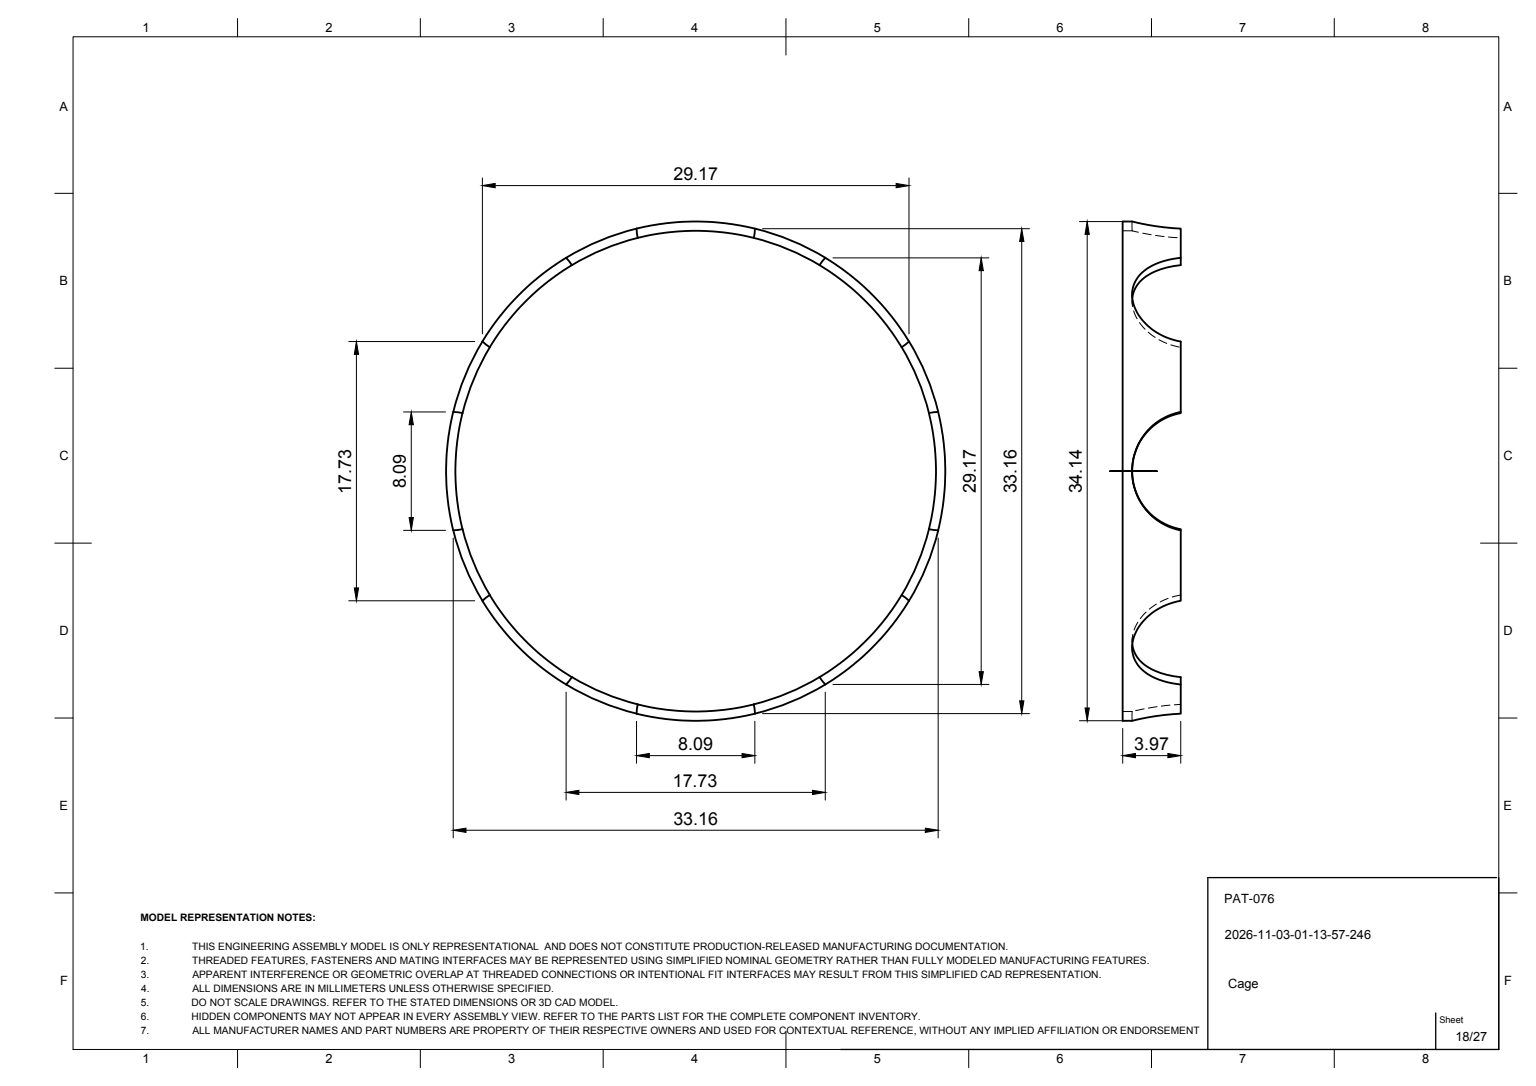
ISO-10303-21;
HEADER;
/* Generated by software containing ST-Developer
 * from STEP Tools, Inc. (www.steptools.com) 
 */

FILE_DESCRIPTION(
/* description */ ('Overhung pulley bearing cartridge'),
/* implementation_level */ '2;1');

FILE_NAME(
/* name */ 'Cage.step',
/* time_stamp */ '2026-10-28T03:22:33-07:00',
/* author */ (''),
/* organization */ (''),
/* preprocessor_version */ 'ST-DEVELOPER v20.2',
/* originating_system */ 'Autodesk Translation Framework v15.17.0.0',
/* authorisation */ '');

FILE_SCHEMA (('AUTOMOTIVE_DESIGN { 1 0 10303 214 3 1 1 }'));
ENDSEC;

DATA;
#10=MECHANICAL_DESIGN_GEOMETRIC_PRESENTATION_REPRESENTATION('',(#301),#10963);
#163=B_SPLINE_CURVE_WITH_KNOTS('',3,(#9085,#9086,#9087,#9088,#9089,#9090,
#9091,#9092,#9093,#9094,#9095,#9096,#9097,#9098,#9099,#9100,#9101,#9102,
#9103,#9104,#9105,#9106),.UNSPECIFIED.,.F.,.F.,(4,2,2,2,2,2,2,2,2,2,4),
(0.0789094028588958,0.210573405340968,0.315860108011452,0.421146810681936,
0.522142632548711,0.623138454415485,0.72413427628226,0.825130098149035,
0.930416800819519,1.03570350349,1.16736750597208),.UNSPECIFIED.);
#164=B_SPLINE_CURVE_WITH_KNOTS('',3,(#9110,#9111,#9112,#9113,#9114,#9115,
#9116,#9117,#9118,#9119,#9120,#9121,#9122,#9123,#9124,#9125,#9126,#9127,
#9128,#9129,#9130,#9131),.UNSPECIFIED.,.F.,.F.,(4,2,2,2,2,2,2,2,2,2,4),
(0.0774793363974613,0.142088896491891,0.284177792983782,0.411119756996526,
0.514392970548519,0.617666184100513,0.720939397652506,0.8242126112045,0.951154575217244,
1.09324347170913,1.15785303180356),.UNSPECIFIED.);
#165=B_SPLINE_CURVE_WITH_KNOTS('',3,(#9137,#9138,#9139,#9140,#9141,#9142,
#9143,#9144,#9145,#9146,#9147,#9148,#9149,#9150,#9151,#9152,#9153,#9154,
#9155,#9156,#9157,#9158),.UNSPECIFIED.,.F.,.F.,(4,2,2,2,2,2,2,2,2,2,4),
(0.0774793363974613,0.142088896491891,0.284177792983782,0.411119756996525,
0.514392970548519,0.617666184100513,0.720939397652506,0.8242126112045,0.951154575217243,
1.09324347170913,1.15785303180356),.UNSPECIFIED.);
#166=B_SPLINE_CURVE_WITH_KNOTS('',3,(#9162,#9163,#9164,#9165,#9166,#9167,
#9168,#9169,#9170,#9171,#9172,#9173,#9174,#9175,#9176,#9177,#9178,#9179,
#9180,#9181,#9182,#9183),.UNSPECIFIED.,.F.,.F.,(4,2,2,2,2,2,2,2,2,2,4),
(0.0774793363974614,0.142088896491891,0.284177792983781,0.411119756996525,
0.514392970548519,0.617666184100512,0.720939397652506,0.824212611204499,
0.951154575217243,1.09324347170913,1.15785303180356),.UNSPECIFIED.);
#167=B_SPLINE_CURVE_WITH_KNOTS('',3,(#9187,#9188,#9189,#9190,#9191,#9192,
#9193,#9194,#9195,#9196,#9197,#9198),.UNSPECIFIED.,.F.,.F.,(4,2,2,2,2,4),
(0.0774793363974613,0.142088896491891,0.284177792983781,0.411119756996525,
0.514392970548519,0.617666184100512),.UNSPECIFIED.);
#168=B_SPLINE_CURVE_WITH_KNOTS('',3,(#9203,#9204,#9205,#9206,#9207,#9208,
#9209,#9210,#9211,#9212,#9213,#9214),.UNSPECIFIED.,.F.,.F.,(4,2,2,2,2,4),
(0.617666184100512,0.720939397652506,0.824212611204499,0.951154575217243,
1.09324347170913,1.15785303180356),.UNSPECIFIED.);
#169=B_SPLINE_CURVE_WITH_KNOTS('',3,(#9218,#9219,#9220,#9221,#9222,#9223,
#9224,#9225,#9226,#9227,#9228,#9229,#9230,#9231,#9232,#9233,#9234,#9235,
#9236,#9237,#9238,#9239),.UNSPECIFIED.,.F.,.F.,(4,2,2,2,2,2,2,2,2,2,4),
(0.0774793363974613,0.142088896491891,0.284177792983782,0.411119756996526,
0.514392970548519,0.617666184100513,0.720939397652507,0.8242126112045,0.951154575217245,
1.09324347170914,1.15785303180356),.UNSPECIFIED.);
#170=B_SPLINE_CURVE_WITH_KNOTS('',3,(#9243,#9244,#9245,#9246,#9247,#9248,
#9249,#9250,#9251,#9252,#9253,#9254,#9255,#9256,#9257,#9258,#9259,#9260,
#9261,#9262,#9263,#9264),.UNSPECIFIED.,.F.,.F.,(4,2,2,2,2,2,2,2,2,2,4),
(0.0774793363974613,0.142088896491891,0.284177792983782,0.411119756996526,
0.514392970548519,0.617666184100513,0.720939397652506,0.824212611204499,
0.951154575217243,1.09324347170913,1.15785303180356),.UNSPECIFIED.);
#171=B_SPLINE_CURVE_WITH_KNOTS('',3,(#9268,#9269,#9270,#9271,#9272,#9273,
#9274,#9275,#9276,#9277,#9278,#9279,#9280,#9281,#9282,#9283,#9284,#9285,
#9286,#9287,#9288,#9289),.UNSPECIFIED.,.F.,.F.,(4,2,2,2,2,2,2,2,2,2,4),
(0.0774793363974613,0.142088896491891,0.284177792983782,0.411119756996526,
0.514392970548519,0.617666184100513,0.720939397652506,0.8242126112045,0.951154575217244,
1.09324347170913,1.15785303180356),.UNSPECIFIED.);
#172=B_SPLINE_CURVE_WITH_KNOTS('',3,(#9293,#9294,#9295,#9296,#9297,#9298,
#9299,#9300,#9301,#9302,#9303,#9304,#9305,#9306,#9307,#9308,#9309,#9310,
#9311,#9312,#9313,#9314),.UNSPECIFIED.,.F.,.F.,(4,2,2,2,2,2,2,2,2,2,4),
(0.0774793363974613,0.142088896491891,0.284177792983782,0.411119756996526,
0.514392970548519,0.617666184100513,0.720939397652506,0.8242126112045,0.951154575217243,
1.09324347170913,1.15785303180356),.UNSPECIFIED.);
#173=B_SPLINE_CURVE_WITH_KNOTS('',3,(#9322,#9323,#9324,#9325,#9326,#9327,
#9328,#9329,#9330,#9331,#9332,#9333,#9334,#9335,#9336,#9337,#9338,#9339,
#9340,#9341,#9342,#9343),.UNSPECIFIED.,.F.,.F.,(4,2,2,2,2,2,2,2,2,2,4),
(0.0789094028588958,0.210573405340968,0.315860108011452,0.421146810681936,
0.522142632548711,0.623138454415485,0.72413427628226,0.825130098149035,
0.930416800819519,1.03570350349,1.16736750597208),.UNSPECIFIED.);
#174=B_SPLINE_CURVE_WITH_KNOTS('',3,(#9351,#9352,#9353,#9354,#9355,#9356,
#9357,#9358,#9359,#9360,#9361,#9362,#9363,#9364,#9365,#9366,#9367,#9368,
#9369,#9370,#9371,#9372),.UNSPECIFIED.,.F.,.F.,(4,2,2,2,2,2,2,2,2,2,4),
(0.0789094028588958,0.210573405340969,0.315860108011453,0.421146810681937,
0.522142632548712,0.623138454415486,0.724134276282261,0.825130098149035,
0.930416800819519,1.03570350349,1.16736750597208),.UNSPECIFIED.);
#175=B_SPLINE_CURVE_WITH_KNOTS('',3,(#9381,#9382,#9383,#9384,#9385,#9386,
#9387,#9388,#9389,#9390,#9391,#9392),.UNSPECIFIED.,.F.,.F.,(4,2,2,2,2,4),
(0.0789094028588958,0.210573405340968,0.315860108011452,0.421146810681937,
0.522142632548711,0.623138454415486),.UNSPECIFIED.);
#176=B_SPLINE_CURVE_WITH_KNOTS('',3,(#9394,#9395,#9396,#9397,#9398,#9399,
#9400,#9401,#9402,#9403,#9404,#9405),.UNSPECIFIED.,.F.,.F.,(4,2,2,2,2,4),
(0.623138454415486,0.72413427628226,0.825130098149035,0.930416800819519,
1.03570350349,1.16736750597208),.UNSPECIFIED.);
#177=B_SPLINE_CURVE_WITH_KNOTS('',3,(#9412,#9413,#9414,#9415,#9416,#9417,
#9418,#9419,#9420,#9421,#9422,#9423,#9424,#9425,#9426,#9427,#9428,#9429,
#9430,#9431,#9432,#9433),.UNSPECIFIED.,.F.,.F.,(4,2,2,2,2,2,2,2,2,2,4),
(0.0789094028588958,0.210573405340968,0.315860108011452,0.421146810681936,
0.522142632548711,0.623138454415486,0.72413427628226,0.825130098149035,
0.930416800819519,1.03570350349,1.16736750597208),.UNSPECIFIED.);
#178=B_SPLINE_CURVE_WITH_KNOTS('',3,(#9441,#9442,#9443,#9444,#9445,#9446,
#9447,#9448,#9449,#9450,#9451,#9452,#9453,#9454,#9455,#9456,#9457,#9458,
#9459,#9460,#9461,#9462),.UNSPECIFIED.,.F.,.F.,(4,2,2,2,2,2,2,2,2,2,4),
(0.0789094028588957,0.210573405340968,0.315860108011452,0.421146810681936,
0.522142632548711,0.623138454415485,0.72413427628226,0.825130098149035,
0.930416800819519,1.03570350349,1.16736750597207),.UNSPECIFIED.);
#179=B_SPLINE_CURVE_WITH_KNOTS('',3,(#9470,#9471,#9472,#9473,#9474,#9475,
#9476,#9477,#9478,#9479,#9480,#9481,#9482,#9483,#9484,#9485,#9486,#9487,
#9488,#9489,#9490,#9491),.UNSPECIFIED.,.F.,.F.,(4,2,2,2,2,2,2,2,2,2,4),
(0.0789094028588958,0.210573405340968,0.315860108011452,0.421146810681936,
0.522142632548711,0.623138454415486,0.72413427628226,0.825130098149035,
0.930416800819519,1.03570350349,1.16736750597208),.UNSPECIFIED.);
#180=B_SPLINE_CURVE_WITH_KNOTS('',3,(#9500,#9501,#9502,#9503,#9504,#9505,
#9506,#9507,#9508,#9509,#9510,#9511,#9512,#9513,#9514,#9515,#9516,#9517,
#9518,#9519,#9520,#9521),.UNSPECIFIED.,.F.,.F.,(4,2,2,2,2,2,2,2,2,2,4),
(0.0789094028588958,0.210573405340968,0.315860108011452,0.421146810681936,
0.522142632548711,0.623138454415485,0.72413427628226,0.825130098149035,
0.930416800819519,1.03570350349,1.16736750597208),.UNSPECIFIED.);
#215=SPHERICAL_SURFACE('',#6170,0.412776);
#216=SPHERICAL_SURFACE('',#6186,0.412776);
#217=SPHERICAL_SURFACE('',#6191,0.412776);
#218=SPHERICAL_SURFACE('',#6196,0.412776);
#219=SPHERICAL_SURFACE('',#6201,0.412776);
#220=SPHERICAL_SURFACE('',#6206,0.412776);
#221=SPHERICAL_SURFACE('',#6211,0.412776);
#222=SPHERICAL_SURFACE('',#6219,0.412776);
#250=SHAPE_REPRESENTATION_RELATIONSHIP('SRR','None',#11071,#272);
#272=ADVANCED_BREP_SHAPE_REPRESENTATION('',(#331),#10951);
#301=STYLED_ITEM('',(#11253),#331);
#331=MANIFOLD_SOLID_BREP('Continuous crown cage',#5668);
#400=FACE_BOUND('',#1101,.T.);
#495=PLANE('',#6183);
#496=PLANE('',#6188);
#497=PLANE('',#6193);
#498=PLANE('',#6198);
#499=PLANE('',#6203);
#500=PLANE('',#6208);
#501=PLANE('',#6217);
#502=PLANE('',#6221);
#503=PLANE('',#6222);
#695=FACE_OUTER_BOUND('',#1083,.T.);
#696=FACE_OUTER_BOUND('',#1084,.T.);
#697=FACE_OUTER_BOUND('',#1085,.T.);
#698=FACE_OUTER_BOUND('',#1086,.T.);
#699=FACE_OUTER_BOUND('',#1087,.T.);
#700=FACE_OUTER_BOUND('',#1088,.T.);
#701=FACE_OUTER_BOUND('',#1089,.T.);
#702=FACE_OUTER_BOUND('',#1090,.T.);
#703=FACE_OUTER_BOUND('',#1091,.T.);
#704=FACE_OUTER_BOUND('',#1092,.T.);
#705=FACE_OUTER_BOUND('',#1093,.T.);
#706=FACE_OUTER_BOUND('',#1094,.T.);
#707=FACE_OUTER_BOUND('',#1095,.T.);
#708=FACE_OUTER_BOUND('',#1096,.T.);
#709=FACE_OUTER_BOUND('',#1097,.T.);
#710=FACE_OUTER_BOUND('',#1098,.T.);
#711=FACE_OUTER_BOUND('',#1099,.T.);
#712=FACE_OUTER_BOUND('',#1100,.T.);
#713=FACE_OUTER_BOUND('',#1102,.T.);
#1083=EDGE_LOOP('',(#4115,#4116,#4117,#4118));
#1084=EDGE_LOOP('',(#4119,#4120,#4121,#4122,#4123,#4124,#4125,#4126,#4127,
#4128,#4129,#4130,#4131,#4132,#4133,#4134,#4135,#4136,#4137,#4138));
#1085=EDGE_LOOP('',(#4139,#4140,#4141,#4142));
#1086=EDGE_LOOP('',(#4143,#4144,#4145,#4146));
#1087=EDGE_LOOP('',(#4147,#4148,#4149,#4150));
#1088=EDGE_LOOP('',(#4151,#4152,#4153,#4154));
#1089=EDGE_LOOP('',(#4155,#4156,#4157,#4158));
#1090=EDGE_LOOP('',(#4159,#4160,#4161,#4162,#4163,#4164));
#1091=EDGE_LOOP('',(#4165,#4166,#4167,#4168));
#1092=EDGE_LOOP('',(#4169,#4170,#4171,#4172));
#1093=EDGE_LOOP('',(#4173,#4174,#4175,#4176));
#1094=EDGE_LOOP('',(#4177,#4178,#4179,#4180));
#1095=EDGE_LOOP('',(#4181,#4182,#4183,#4184));
#1096=EDGE_LOOP('',(#4185,#4186,#4187,#4188));
#1097=EDGE_LOOP('',(#4189,#4190,#4191,#4192,#4193,#4194,#4195,#4196,#4197,
#4198,#4199,#4200,#4201,#4202,#4203,#4204,#4205,#4206,#4207,#4208));
#1098=EDGE_LOOP('',(#4209,#4210,#4211,#4212));
#1099=EDGE_LOOP('',(#4213,#4214,#4215,#4216));
#1100=EDGE_LOOP('',(#4217));
#1101=EDGE_LOOP('',(#4218));
#1102=EDGE_LOOP('',(#4219,#4220,#4221,#4222));
#1447=LINE('',#9200,#1789);
#1448=LINE('',#9496,#1790);
#1789=VECTOR('',#7311,1.706752);
#1790=VECTOR('',#7388,1.643248);
#2124=CIRCLE('',#6171,0.405071403305639);
#2125=CIRCLE('',#6172,0.405071403305639);
#2126=CIRCLE('',#6174,1.706752);
#2127=CIRCLE('',#6175,1.706752);
#2128=CIRCLE('',#6176,1.706752);
#2129=CIRCLE('',#6177,1.706752);
#2130=CIRCLE('',#6178,1.706752);
#2131=CIRCLE('',#6179,1.706752);
#2132=CIRCLE('',#6180,1.706752);
#2133=CIRCLE('',#6181,1.706752);
#2134=CIRCLE('',#6182,1.706752);
#2135=CIRCLE('',#6184,1.643248);
#2136=CIRCLE('',#6185,0.405071403305639);
#2137=CIRCLE('',#6187,0.405071403305639);
#2138=CIRCLE('',#6189,1.643248);
#2139=CIRCLE('',#6190,0.405071403305639);
#2140=CIRCLE('',#6192,0.405071403305639);
#2141=CIRCLE('',#6194,1.643248);
#2142=CIRCLE('',#6195,0.405071403305639);
#2143=CIRCLE('',#6197,0.405071403305639);
#2144=CIRCLE('',#6199,1.643248);
#2145=CIRCLE('',#6200,0.405071403305639);
#2146=CIRCLE('',#6202,0.405071403305639);
#2147=CIRCLE('',#6204,1.643248);
#2148=CIRCLE('',#6205,0.405071403305639);
#2149=CIRCLE('',#6207,0.405071403305639);
#2150=CIRCLE('',#6209,1.643248);
#2151=CIRCLE('',#6210,0.405071403305639);
#2152=CIRCLE('',#6212,0.405071403305639);
#2153=CIRCLE('',#6214,1.643248);
#2154=CIRCLE('',#6215,1.643248);
#2155=CIRCLE('',#6216,1.643248);
#2156=CIRCLE('',#6218,0.405071403305639);
#2157=CIRCLE('',#6220,0.405071403305639);
#2545=VERTEX_POINT('',#9083);
#2546=VERTEX_POINT('',#9084);
#2547=VERTEX_POINT('',#9107);
#2548=VERTEX_POINT('',#9109);
#2549=VERTEX_POINT('',#9134);
#2550=VERTEX_POINT('',#9136);
#2551=VERTEX_POINT('',#9159);
#2552=VERTEX_POINT('',#9161);
#2553=VERTEX_POINT('',#9184);
#2554=VERTEX_POINT('',#9186);
#2555=VERTEX_POINT('',#9199);
#2556=VERTEX_POINT('',#9202);
#2557=VERTEX_POINT('',#9215);
#2558=VERTEX_POINT('',#9217);
#2559=VERTEX_POINT('',#9240);
#2560=VERTEX_POINT('',#9242);
#2561=VERTEX_POINT('',#9265);
#2562=VERTEX_POINT('',#9267);
#2563=VERTEX_POINT('',#9290);
#2564=VERTEX_POINT('',#9292);
#2565=VERTEX_POINT('',#9317);
#2566=VERTEX_POINT('',#9321);
#2567=VERTEX_POINT('',#9346);
#2568=VERTEX_POINT('',#9350);
#2569=VERTEX_POINT('',#9375);
#2570=VERTEX_POINT('',#9379);
#2571=VERTEX_POINT('',#9380);
#2572=VERTEX_POINT('',#9407);
#2573=VERTEX_POINT('',#9411);
#2574=VERTEX_POINT('',#9436);
#2575=VERTEX_POINT('',#9440);
#2576=VERTEX_POINT('',#9465);
#2577=VERTEX_POINT('',#9469);
#2578=VERTEX_POINT('',#9494);
#2579=VERTEX_POINT('',#9497);
#2580=VERTEX_POINT('',#9499);
#3127=EDGE_CURVE('',#2545,#2546,#163,.T.);
#3128=EDGE_CURVE('',#2547,#2545,#2124,.T.);
#3129=EDGE_CURVE('',#2548,#2547,#164,.T.);
#3130=EDGE_CURVE('',#2546,#2548,#2125,.T.);
#3131=EDGE_CURVE('',#2549,#2547,#2126,.T.);
#3132=EDGE_CURVE('',#2549,#2550,#165,.T.);
#3133=EDGE_CURVE('',#2551,#2550,#2127,.T.);
#3134=EDGE_CURVE('',#2551,#2552,#166,.T.);
#3135=EDGE_CURVE('',#2553,#2552,#2128,.T.);
#3136=EDGE_CURVE('',#2553,#2554,#167,.T.);
#3137=EDGE_CURVE('',#2554,#2555,#1447,.T.);
#3138=EDGE_CURVE('',#2555,#2555,#2129,.T.);
#3139=EDGE_CURVE('',#2554,#2556,#168,.T.);
#3140=EDGE_CURVE('',#2557,#2556,#2130,.T.);
#3141=EDGE_CURVE('',#2557,#2558,#169,.T.);
#3142=EDGE_CURVE('',#2559,#2558,#2131,.T.);
#3143=EDGE_CURVE('',#2559,#2560,#170,.T.);
#3144=EDGE_CURVE('',#2561,#2560,#2132,.T.);
#3145=EDGE_CURVE('',#2561,#2562,#171,.T.);
#3146=EDGE_CURVE('',#2563,#2562,#2133,.T.);
#3147=EDGE_CURVE('',#2563,#2564,#172,.T.);
#3148=EDGE_CURVE('',#2548,#2564,#2134,.T.);
#3149=EDGE_CURVE('',#2545,#2565,#2135,.T.);
#3150=EDGE_CURVE('',#2565,#2549,#2136,.T.);
#3151=EDGE_CURVE('',#2566,#2565,#173,.T.);
#3152=EDGE_CURVE('',#2550,#2566,#2137,.T.);
#3153=EDGE_CURVE('',#2566,#2567,#2138,.T.);
#3154=EDGE_CURVE('',#2567,#2551,#2139,.T.);
#3155=EDGE_CURVE('',#2568,#2567,#174,.T.);
#3156=EDGE_CURVE('',#2552,#2568,#2140,.T.);
#3157=EDGE_CURVE('',#2568,#2569,#2141,.T.);
#3158=EDGE_CURVE('',#2569,#2553,#2142,.T.);
#3159=EDGE_CURVE('',#2570,#2571,#175,.T.);
#3160=EDGE_CURVE('',#2556,#2570,#2143,.T.);
#3161=EDGE_CURVE('',#2571,#2569,#176,.T.);
#3162=EDGE_CURVE('',#2570,#2572,#2144,.T.);
#3163=EDGE_CURVE('',#2572,#2557,#2145,.T.);
#3164=EDGE_CURVE('',#2573,#2572,#177,.T.);
#3165=EDGE_CURVE('',#2558,#2573,#2146,.T.);
#3166=EDGE_CURVE('',#2573,#2574,#2147,.T.);
#3167=EDGE_CURVE('',#2574,#2559,#2148,.T.);
#3168=EDGE_CURVE('',#2575,#2574,#178,.T.);
#3169=EDGE_CURVE('',#2560,#2575,#2149,.T.);
#3170=EDGE_CURVE('',#2575,#2576,#2150,.T.);
#3171=EDGE_CURVE('',#2576,#2561,#2151,.T.);
#3172=EDGE_CURVE('',#2577,#2576,#179,.T.);
#3173=EDGE_CURVE('',#2562,#2577,#2152,.T.);
#3174=EDGE_CURVE('',#2578,#2578,#2153,.T.);
#3175=EDGE_CURVE('',#2578,#2571,#1448,.T.);
#3176=EDGE_CURVE('',#2579,#2546,#2154,.T.);
#3177=EDGE_CURVE('',#2579,#2580,#180,.T.);
#3178=EDGE_CURVE('',#2577,#2580,#2155,.T.);
#3179=EDGE_CURVE('',#2564,#2579,#2156,.T.);
#3180=EDGE_CURVE('',#2580,#2563,#2157,.T.);
#4115=ORIENTED_EDGE('',*,*,#3127,.F.);
#4116=ORIENTED_EDGE('',*,*,#3128,.F.);
#4117=ORIENTED_EDGE('',*,*,#3129,.F.);
#4118=ORIENTED_EDGE('',*,*,#3130,.F.);
#4119=ORIENTED_EDGE('',*,*,#3129,.T.);
#4120=ORIENTED_EDGE('',*,*,#3131,.F.);
#4121=ORIENTED_EDGE('',*,*,#3132,.T.);
#4122=ORIENTED_EDGE('',*,*,#3133,.F.);
#4123=ORIENTED_EDGE('',*,*,#3134,.T.);
#4124=ORIENTED_EDGE('',*,*,#3135,.F.);
#4125=ORIENTED_EDGE('',*,*,#3136,.T.);
#4126=ORIENTED_EDGE('',*,*,#3137,.T.);
#4127=ORIENTED_EDGE('',*,*,#3138,.F.);
#4128=ORIENTED_EDGE('',*,*,#3137,.F.);
#4129=ORIENTED_EDGE('',*,*,#3139,.T.);
#4130=ORIENTED_EDGE('',*,*,#3140,.F.);
#4131=ORIENTED_EDGE('',*,*,#3141,.T.);
#4132=ORIENTED_EDGE('',*,*,#3142,.F.);
#4133=ORIENTED_EDGE('',*,*,#3143,.T.);
#4134=ORIENTED_EDGE('',*,*,#3144,.F.);
#4135=ORIENTED_EDGE('',*,*,#3145,.T.);
#4136=ORIENTED_EDGE('',*,*,#3146,.F.);
#4137=ORIENTED_EDGE('',*,*,#3147,.T.);
#4138=ORIENTED_EDGE('',*,*,#3148,.F.);
#4139=ORIENTED_EDGE('',*,*,#3128,.T.);
#4140=ORIENTED_EDGE('',*,*,#3149,.T.);
#4141=ORIENTED_EDGE('',*,*,#3150,.T.);
#4142=ORIENTED_EDGE('',*,*,#3131,.T.);
#4143=ORIENTED_EDGE('',*,*,#3151,.F.);
#4144=ORIENTED_EDGE('',*,*,#3152,.F.);
#4145=ORIENTED_EDGE('',*,*,#3132,.F.);
#4146=ORIENTED_EDGE('',*,*,#3150,.F.);
#4147=ORIENTED_EDGE('',*,*,#3152,.T.);
#4148=ORIENTED_EDGE('',*,*,#3153,.T.);
#4149=ORIENTED_EDGE('',*,*,#3154,.T.);
#4150=ORIENTED_EDGE('',*,*,#3133,.T.);
#4151=ORIENTED_EDGE('',*,*,#3155,.F.);
#4152=ORIENTED_EDGE('',*,*,#3156,.F.);
#4153=ORIENTED_EDGE('',*,*,#3134,.F.);
#4154=ORIENTED_EDGE('',*,*,#3154,.F.);
#4155=ORIENTED_EDGE('',*,*,#3156,.T.);
#4156=ORIENTED_EDGE('',*,*,#3157,.T.);
#4157=ORIENTED_EDGE('',*,*,#3158,.T.);
#4158=ORIENTED_EDGE('',*,*,#3135,.T.);
#4159=ORIENTED_EDGE('',*,*,#3159,.F.);
#4160=ORIENTED_EDGE('',*,*,#3160,.F.);
#4161=ORIENTED_EDGE('',*,*,#3139,.F.);
#4162=ORIENTED_EDGE('',*,*,#3136,.F.);
#4163=ORIENTED_EDGE('',*,*,#3158,.F.);
#4164=ORIENTED_EDGE('',*,*,#3161,.F.);
#4165=ORIENTED_EDGE('',*,*,#3160,.T.);
#4166=ORIENTED_EDGE('',*,*,#3162,.T.);
#4167=ORIENTED_EDGE('',*,*,#3163,.T.);
#4168=ORIENTED_EDGE('',*,*,#3140,.T.);
#4169=ORIENTED_EDGE('',*,*,#3164,.F.);
#4170=ORIENTED_EDGE('',*,*,#3165,.F.);
#4171=ORIENTED_EDGE('',*,*,#3141,.F.);
#4172=ORIENTED_EDGE('',*,*,#3163,.F.);
#4173=ORIENTED_EDGE('',*,*,#3165,.T.);
#4174=ORIENTED_EDGE('',*,*,#3166,.T.);
#4175=ORIENTED_EDGE('',*,*,#3167,.T.);
#4176=ORIENTED_EDGE('',*,*,#3142,.T.);
#4177=ORIENTED_EDGE('',*,*,#3168,.F.);
#4178=ORIENTED_EDGE('',*,*,#3169,.F.);
#4179=ORIENTED_EDGE('',*,*,#3143,.F.);
#4180=ORIENTED_EDGE('',*,*,#3167,.F.);
#4181=ORIENTED_EDGE('',*,*,#3169,.T.);
#4182=ORIENTED_EDGE('',*,*,#3170,.T.);
#4183=ORIENTED_EDGE('',*,*,#3171,.T.);
#4184=ORIENTED_EDGE('',*,*,#3144,.T.);
#4185=ORIENTED_EDGE('',*,*,#3145,.F.);
#4186=ORIENTED_EDGE('',*,*,#3171,.F.);
#4187=ORIENTED_EDGE('',*,*,#3172,.F.);
#4188=ORIENTED_EDGE('',*,*,#3173,.F.);
#4189=ORIENTED_EDGE('',*,*,#3174,.F.);
#4190=ORIENTED_EDGE('',*,*,#3175,.T.);
#4191=ORIENTED_EDGE('',*,*,#3161,.T.);
#4192=ORIENTED_EDGE('',*,*,#3157,.F.);
#4193=ORIENTED_EDGE('',*,*,#3155,.T.);
#4194=ORIENTED_EDGE('',*,*,#3153,.F.);
#4195=ORIENTED_EDGE('',*,*,#3151,.T.);
#4196=ORIENTED_EDGE('',*,*,#3149,.F.);
#4197=ORIENTED_EDGE('',*,*,#3127,.T.);
#4198=ORIENTED_EDGE('',*,*,#3176,.F.);
#4199=ORIENTED_EDGE('',*,*,#3177,.T.);
#4200=ORIENTED_EDGE('',*,*,#3178,.F.);
#4201=ORIENTED_EDGE('',*,*,#3172,.T.);
#4202=ORIENTED_EDGE('',*,*,#3170,.F.);
#4203=ORIENTED_EDGE('',*,*,#3168,.T.);
#4204=ORIENTED_EDGE('',*,*,#3166,.F.);
#4205=ORIENTED_EDGE('',*,*,#3164,.T.);
#4206=ORIENTED_EDGE('',*,*,#3162,.F.);
#4207=ORIENTED_EDGE('',*,*,#3159,.T.);
#4208=ORIENTED_EDGE('',*,*,#3175,.F.);
#4209=ORIENTED_EDGE('',*,*,#3130,.T.);
#4210=ORIENTED_EDGE('',*,*,#3148,.T.);
#4211=ORIENTED_EDGE('',*,*,#3179,.T.);
#4212=ORIENTED_EDGE('',*,*,#3176,.T.);
#4213=ORIENTED_EDGE('',*,*,#3147,.F.);
#4214=ORIENTED_EDGE('',*,*,#3180,.F.);
#4215=ORIENTED_EDGE('',*,*,#3177,.F.);
#4216=ORIENTED_EDGE('',*,*,#3179,.F.);
#4217=ORIENTED_EDGE('',*,*,#3138,.T.);
#4218=ORIENTED_EDGE('',*,*,#3174,.T.);
#4219=ORIENTED_EDGE('',*,*,#3173,.T.);
#4220=ORIENTED_EDGE('',*,*,#3178,.T.);
#4221=ORIENTED_EDGE('',*,*,#3180,.T.);
#4222=ORIENTED_EDGE('',*,*,#3146,.T.);
#5210=CYLINDRICAL_SURFACE('',#6173,1.706752);
#5211=CYLINDRICAL_SURFACE('',#6213,1.643248);
#5439=ADVANCED_FACE('',(#695),#215,.F.);
#5440=ADVANCED_FACE('',(#696),#5210,.T.);
#5441=ADVANCED_FACE('',(#697),#495,.T.);
#5442=ADVANCED_FACE('',(#698),#216,.F.);
#5443=ADVANCED_FACE('',(#699),#496,.T.);
#5444=ADVANCED_FACE('',(#700),#217,.F.);
#5445=ADVANCED_FACE('',(#701),#497,.T.);
#5446=ADVANCED_FACE('',(#702),#218,.F.);
#5447=ADVANCED_FACE('',(#703),#498,.T.);
#5448=ADVANCED_FACE('',(#704),#219,.F.);
#5449=ADVANCED_FACE('',(#705),#499,.T.);
#5450=ADVANCED_FACE('',(#706),#220,.F.);
#5451=ADVANCED_FACE('',(#707),#500,.T.);
#5452=ADVANCED_FACE('',(#708),#221,.F.);
#5453=ADVANCED_FACE('',(#709),#5211,.F.);
#5454=ADVANCED_FACE('',(#710),#501,.T.);
#5455=ADVANCED_FACE('',(#711),#222,.F.);
#5456=ADVANCED_FACE('',(#712,#400),#502,.T.);
#5457=ADVANCED_FACE('',(#713),#503,.T.);
#5668=CLOSED_SHELL('',(#5439,#5440,#5441,#5442,#5443,#5444,#5445,#5446,
#5447,#5448,#5449,#5450,#5451,#5452,#5453,#5454,#5455,#5456,#5457));
#6169=AXIS2_PLACEMENT_3D('',#9081,#7295,#7296);
#6170=AXIS2_PLACEMENT_3D('',#9082,#7297,#7298);
#6171=AXIS2_PLACEMENT_3D('',#9108,#7299,#7300);
#6172=AXIS2_PLACEMENT_3D('',#9132,#7301,#7302);
#6173=AXIS2_PLACEMENT_3D('',#9133,#7303,#7304);
#6174=AXIS2_PLACEMENT_3D('',#9135,#7305,#7306);
#6175=AXIS2_PLACEMENT_3D('',#9160,#7307,#7308);
#6176=AXIS2_PLACEMENT_3D('',#9185,#7309,#7310);
#6177=AXIS2_PLACEMENT_3D('',#9201,#7312,#7313);
#6178=AXIS2_PLACEMENT_3D('',#9216,#7314,#7315);
#6179=AXIS2_PLACEMENT_3D('',#9241,#7316,#7317);
#6180=AXIS2_PLACEMENT_3D('',#9266,#7318,#7319);
#6181=AXIS2_PLACEMENT_3D('',#9291,#7320,#7321);
#6182=AXIS2_PLACEMENT_3D('',#9315,#7322,#7323);
#6183=AXIS2_PLACEMENT_3D('',#9316,#7324,#7325);
#6184=AXIS2_PLACEMENT_3D('',#9318,#7326,#7327);
#6185=AXIS2_PLACEMENT_3D('',#9319,#7328,#7329);
#6186=AXIS2_PLACEMENT_3D('',#9320,#7330,#7331);
#6187=AXIS2_PLACEMENT_3D('',#9344,#7332,#7333);
#6188=AXIS2_PLACEMENT_3D('',#9345,#7334,#7335);
#6189=AXIS2_PLACEMENT_3D('',#9347,#7336,#7337);
#6190=AXIS2_PLACEMENT_3D('',#9348,#7338,#7339);
#6191=AXIS2_PLACEMENT_3D('',#9349,#7340,#7341);
#6192=AXIS2_PLACEMENT_3D('',#9373,#7342,#7343);
#6193=AXIS2_PLACEMENT_3D('',#9374,#7344,#7345);
#6194=AXIS2_PLACEMENT_3D('',#9376,#7346,#7347);
#6195=AXIS2_PLACEMENT_3D('',#9377,#7348,#7349);
#6196=AXIS2_PLACEMENT_3D('',#9378,#7350,#7351);
#6197=AXIS2_PLACEMENT_3D('',#9393,#7352,#7353);
#6198=AXIS2_PLACEMENT_3D('',#9406,#7354,#7355);
#6199=AXIS2_PLACEMENT_3D('',#9408,#7356,#7357);
#6200=AXIS2_PLACEMENT_3D('',#9409,#7358,#7359);
#6201=AXIS2_PLACEMENT_3D('',#9410,#7360,#7361);
#6202=AXIS2_PLACEMENT_3D('',#9434,#7362,#7363);
#6203=AXIS2_PLACEMENT_3D('',#9435,#7364,#7365);
#6204=AXIS2_PLACEMENT_3D('',#9437,#7366,#7367);
#6205=AXIS2_PLACEMENT_3D('',#9438,#7368,#7369);
#6206=AXIS2_PLACEMENT_3D('',#9439,#7370,#7371);
#6207=AXIS2_PLACEMENT_3D('',#9463,#7372,#7373);
#6208=AXIS2_PLACEMENT_3D('',#9464,#7374,#7375);
#6209=AXIS2_PLACEMENT_3D('',#9466,#7376,#7377);
#6210=AXIS2_PLACEMENT_3D('',#9467,#7378,#7379);
#6211=AXIS2_PLACEMENT_3D('',#9468,#7380,#7381);
#6212=AXIS2_PLACEMENT_3D('',#9492,#7382,#7383);
#6213=AXIS2_PLACEMENT_3D('',#9493,#7384,#7385);
#6214=AXIS2_PLACEMENT_3D('',#9495,#7386,#7387);
#6215=AXIS2_PLACEMENT_3D('',#9498,#7389,#7390);
#6216=AXIS2_PLACEMENT_3D('',#9522,#7391,#7392);
#6217=AXIS2_PLACEMENT_3D('',#9523,#7393,#7394);
#6218=AXIS2_PLACEMENT_3D('',#9524,#7395,#7396);
#6219=AXIS2_PLACEMENT_3D('',#9525,#7397,#7398);
#6220=AXIS2_PLACEMENT_3D('',#9526,#7399,#7400);
#6221=AXIS2_PLACEMENT_3D('',#9527,#7401,#7402);
#6222=AXIS2_PLACEMENT_3D('',#9528,#7403,#7404);
#7295=DIRECTION('axis',(0.,0.,1.));
#7296=DIRECTION('refdir',(1.,0.,0.));
#7297=DIRECTION('center_axis',(0.,0.,1.));
#7298=DIRECTION('ref_axis',(1.,0.,0.));
#7299=DIRECTION('center_axis',(0.,-1.,0.));
#7300=DIRECTION('ref_axis',(0.,0.,-1.));
#7301=DIRECTION('center_axis',(0.,-1.,0.));
#7302=DIRECTION('ref_axis',(0.,0.,-1.));
#7303=DIRECTION('center_axis',(0.,1.,0.));
#7304=DIRECTION('ref_axis',(1.,0.,0.));
#7305=DIRECTION('center_axis',(0.,1.,0.));
#7306=DIRECTION('ref_axis',(1.,0.,0.));
#7307=DIRECTION('center_axis',(0.,1.,0.));
#7308=DIRECTION('ref_axis',(1.,0.,0.));
#7309=DIRECTION('center_axis',(0.,1.,0.));
#7310=DIRECTION('ref_axis',(1.,0.,0.));
#7311=DIRECTION('',(0.,-1.,0.));
#7312=DIRECTION('center_axis',(0.,-1.,0.));
#7313=DIRECTION('ref_axis',(1.,0.,0.));
#7314=DIRECTION('center_axis',(0.,1.,0.));
#7315=DIRECTION('ref_axis',(1.,0.,0.));
#7316=DIRECTION('center_axis',(0.,1.,0.));
#7317=DIRECTION('ref_axis',(1.,0.,0.));
#7318=DIRECTION('center_axis',(0.,1.,0.));
#7319=DIRECTION('ref_axis',(1.,0.,0.));
#7320=DIRECTION('center_axis',(0.,1.,0.));
#7321=DIRECTION('ref_axis',(1.,0.,0.));
#7322=DIRECTION('center_axis',(0.,1.,0.));
#7323=DIRECTION('ref_axis',(1.,0.,0.));
#7324=DIRECTION('center_axis',(0.,1.,0.));
#7325=DIRECTION('ref_axis',(1.,0.,0.));
#7326=DIRECTION('center_axis',(0.,-1.,0.));
#7327=DIRECTION('ref_axis',(1.,0.,0.));
#7328=DIRECTION('center_axis',(0.,-1.,0.));
#7329=DIRECTION('ref_axis',(0.,0.,-1.));
#7330=DIRECTION('center_axis',(6.12323399573677E-17,0.,1.));
#7331=DIRECTION('ref_axis',(1.,0.,0.));
#7332=DIRECTION('center_axis',(0.,-1.,0.));
#7333=DIRECTION('ref_axis',(0.,0.,-1.));
#7334=DIRECTION('center_axis',(0.,1.,0.));
#7335=DIRECTION('ref_axis',(1.,0.,0.));
#7336=DIRECTION('center_axis',(0.,-1.,0.));
#7337=DIRECTION('ref_axis',(1.,0.,0.));
#7338=DIRECTION('center_axis',(0.,-1.,0.));
#7339=DIRECTION('ref_axis',(0.,0.,-1.));
#7340=DIRECTION('center_axis',(0.,0.,1.));
#7341=DIRECTION('ref_axis',(1.,0.,0.));
#7342=DIRECTION('center_axis',(0.,-1.,0.));
#7343=DIRECTION('ref_axis',(0.,0.,-1.));
#7344=DIRECTION('center_axis',(0.,1.,0.));
#7345=DIRECTION('ref_axis',(1.,0.,0.));
#7346=DIRECTION('center_axis',(0.,-1.,0.));
#7347=DIRECTION('ref_axis',(1.,0.,0.));
#7348=DIRECTION('center_axis',(0.,-1.,0.));
#7349=DIRECTION('ref_axis',(0.,0.,-1.));
#7350=DIRECTION('center_axis',(0.,0.,1.));
#7351=DIRECTION('ref_axis',(1.,0.,0.));
#7352=DIRECTION('center_axis',(0.,-1.,0.));
#7353=DIRECTION('ref_axis',(0.,0.,-1.));
#7354=DIRECTION('center_axis',(0.,1.,0.));
#7355=DIRECTION('ref_axis',(1.,0.,0.));
#7356=DIRECTION('center_axis',(0.,-1.,0.));
#7357=DIRECTION('ref_axis',(1.,0.,0.));
#7358=DIRECTION('center_axis',(0.,-1.,0.));
#7359=DIRECTION('ref_axis',(0.,0.,-1.));
#7360=DIRECTION('center_axis',(0.,0.,1.));
#7361=DIRECTION('ref_axis',(1.,0.,0.));
#7362=DIRECTION('center_axis',(0.,-1.,0.));
#7363=DIRECTION('ref_axis',(0.,0.,-1.));
#7364=DIRECTION('center_axis',(0.,1.,0.));
#7365=DIRECTION('ref_axis',(1.,0.,0.));
#7366=DIRECTION('center_axis',(0.,-1.,0.));
#7367=DIRECTION('ref_axis',(1.,0.,0.));
#7368=DIRECTION('center_axis',(0.,-1.,0.));
#7369=DIRECTION('ref_axis',(0.,0.,-1.));
#7370=DIRECTION('center_axis',(6.12323399573676E-17,0.,1.));
#7371=DIRECTION('ref_axis',(1.,0.,0.));
#7372=DIRECTION('center_axis',(0.,-1.,0.));
#7373=DIRECTION('ref_axis',(0.,0.,-1.));
#7374=DIRECTION('center_axis',(0.,1.,0.));
#7375=DIRECTION('ref_axis',(1.,0.,0.));
#7376=DIRECTION('center_axis',(0.,-1.,0.));
#7377=DIRECTION('ref_axis',(1.,0.,0.));
#7378=DIRECTION('center_axis',(0.,-1.,0.));
#7379=DIRECTION('ref_axis',(0.,0.,-1.));
#7380=DIRECTION('center_axis',(0.,0.,1.));
#7381=DIRECTION('ref_axis',(1.,0.,0.));
#7382=DIRECTION('center_axis',(0.,-1.,0.));
#7383=DIRECTION('ref_axis',(0.,0.,-1.));
#7384=DIRECTION('center_axis',(0.,1.,0.));
#7385=DIRECTION('ref_axis',(1.,0.,0.));
#7386=DIRECTION('center_axis',(0.,1.,0.));
#7387=DIRECTION('ref_axis',(1.,0.,0.));
#7388=DIRECTION('',(0.,1.,0.));
#7389=DIRECTION('center_axis',(0.,-1.,0.));
#7390=DIRECTION('ref_axis',(1.,0.,0.));
#7391=DIRECTION('center_axis',(0.,-1.,0.));
#7392=DIRECTION('ref_axis',(1.,0.,0.));
#7393=DIRECTION('center_axis',(0.,1.,0.));
#7394=DIRECTION('ref_axis',(1.,0.,0.));
#7395=DIRECTION('center_axis',(0.,-1.,0.));
#7396=DIRECTION('ref_axis',(0.,0.,-1.));
#7397=DIRECTION('center_axis',(0.,0.,1.));
#7398=DIRECTION('ref_axis',(1.,0.,0.));
#7399=DIRECTION('center_axis',(0.,-1.,0.));
#7400=DIRECTION('ref_axis',(0.,0.,-1.));
#7401=DIRECTION('center_axis',(0.,-1.,0.));
#7402=DIRECTION('ref_axis',(-1.,0.,0.));
#7403=DIRECTION('center_axis',(0.,1.,0.));
#7404=DIRECTION('ref_axis',(1.,0.,0.));
#9081=CARTESIAN_POINT('',(0.,0.,0.));
#9082=CARTESIAN_POINT('Origin',(1.18440385848747,0.,1.18440385848747));
#9083=CARTESIAN_POINT('',(0.846804978391753,-0.07938,1.40825612658882));
#9084=CARTESIAN_POINT('',(1.40825612658882,-0.07938,0.846804978391754));
#9085=CARTESIAN_POINT('Ctrl Pts',(0.846804978391752,-0.0793800000000001,
1.40825612658882));
#9086=CARTESIAN_POINT('Ctrl Pts',(0.854205272175554,-0.123401821157026,
1.40380622184538));
#9087=CARTESIAN_POINT('Ctrl Pts',(0.867957148219441,-0.166543350814306,
1.39550172959303));
#9088=CARTESIAN_POINT('Ctrl Pts',(0.902193646979982,-0.237231147975234,
1.3735491215176));
#9089=CARTESIAN_POINT('Ctrl Pts',(0.920778333482564,-0.266264900654909,
1.36127834356734));
#9090=CARTESIAN_POINT('Ctrl Pts',(0.962485392528369,-0.317195968905306,
1.33211611256184));
#9091=CARTESIAN_POINT('Ctrl Pts',(0.985600426557816,-0.33909093068465,1.31521005565926));
#9092=CARTESIAN_POINT('Ctrl Pts',(1.03253285680459,-0.373586846396559,1.27866649102984));
#9093=CARTESIAN_POINT('Ctrl Pts',(1.05871835910697,-0.388086240756494,1.25722555095714));
#9094=CARTESIAN_POINT('Ctrl Pts',(1.11153475808518,-0.407068917407805,1.2107812086231));
#9095=CARTESIAN_POINT('Ctrl Pts',(1.13814686046673,-0.411552957311693,1.18575674747573));
#9096=CARTESIAN_POINT('Ctrl Pts',(1.18575674747573,-0.411552957311693,1.13814686046673));
#9097=CARTESIAN_POINT('Ctrl Pts',(1.2107812086231,-0.407068917407805,1.11153475808518));
#9098=CARTESIAN_POINT('Ctrl Pts',(1.25722555095713,-0.388086240756494,1.05871835910697));
#9099=CARTESIAN_POINT('Ctrl Pts',(1.27866649102984,-0.373586846396559,1.03253285680459));
#9100=CARTESIAN_POINT('Ctrl Pts',(1.31521005565926,-0.33909093068465,0.985600426557816));
#9101=CARTESIAN_POINT('Ctrl Pts',(1.33211611256184,-0.317195968905306,0.962485392528369));
#9102=CARTESIAN_POINT('Ctrl Pts',(1.36127834356734,-0.266264900654909,0.920778333482565));
#9103=CARTESIAN_POINT('Ctrl Pts',(1.3735491215176,-0.237231147975234,0.902193646979983));
#9104=CARTESIAN_POINT('Ctrl Pts',(1.39550172959303,-0.166543350814306,0.867957148219442));
#9105=CARTESIAN_POINT('Ctrl Pts',(1.40380622184538,-0.123401821157026,0.854205272175555));
#9106=CARTESIAN_POINT('Ctrl Pts',(1.40825612658882,-0.0793800000000001,
0.846804978391753));
#9107=CARTESIAN_POINT('',(0.886256117232623,-0.07938,1.45861320581289));
#9108=CARTESIAN_POINT('Origin',(1.18440385848747,-0.07938,1.18440385848747));
#9109=CARTESIAN_POINT('',(1.45861320581289,-0.07938,0.886256117232624));
#9110=CARTESIAN_POINT('Ctrl Pts',(1.45861320581289,-0.0793800000000001,
0.886256117232623));
#9111=CARTESIAN_POINT('Ctrl Pts',(1.45630208793976,-0.101649918886749,0.890059788636852));
#9112=CARTESIAN_POINT('Ctrl Pts',(1.45296717977858,-0.123823518623746,0.895520212222107));
#9113=CARTESIAN_POINT('Ctrl Pts',(1.43904931717599,-0.192480977588836,0.917859913453975));
#9114=CARTESIAN_POINT('Ctrl Pts',(1.4243271592157,-0.236152929235938,0.940896403863072));
#9115=CARTESIAN_POINT('Ctrl Pts',(1.39055359345152,-0.303141259068212,0.990027513266106));
#9116=CARTESIAN_POINT('Ctrl Pts',(1.36743459453896,-0.335108247315849,1.02199477007745));
#9117=CARTESIAN_POINT('Ctrl Pts',(1.32643091652006,-0.373243761060364,1.07446535104584));
#9118=CARTESIAN_POINT('Ctrl Pts',(1.30441816675528,-0.387888272594439,1.10126842659597));
#9119=CARTESIAN_POINT('Ctrl Pts',(1.25681160160691,-0.407041111792943,1.15530234155453));
#9120=CARTESIAN_POINT('Ctrl Pts',(1.23119764287622,-0.411552957311693,1.18251418313119));
#9121=CARTESIAN_POINT('Ctrl Pts',(1.18251418313119,-0.411552957311693,1.23119764287622));
#9122=CARTESIAN_POINT('Ctrl Pts',(1.15530234155453,-0.407041111792943,1.25681160160691));
#9123=CARTESIAN_POINT('Ctrl Pts',(1.10126842659597,-0.387888272594439,1.30441816675528));
#9124=CARTESIAN_POINT('Ctrl Pts',(1.07446535104584,-0.373243761060364,1.32643091652006));
#9125=CARTESIAN_POINT('Ctrl Pts',(1.02199477007745,-0.335108247315848,1.36743459453896));
#9126=CARTESIAN_POINT('Ctrl Pts',(0.990027513266105,-0.303141259068211,
1.39055359345152));
#9127=CARTESIAN_POINT('Ctrl Pts',(0.940896403863071,-0.236152929235937,
1.42432715921571));
#9128=CARTESIAN_POINT('Ctrl Pts',(0.917859913453974,-0.192480977588835,
1.43904931717599));
#9129=CARTESIAN_POINT('Ctrl Pts',(0.895520212222106,-0.123823518623745,
1.45296717977858));
#9130=CARTESIAN_POINT('Ctrl Pts',(0.890059788636851,-0.101649918886749,
1.45630208793976));
#9131=CARTESIAN_POINT('Ctrl Pts',(0.886256117232622,-0.0793800000000001,
1.45861320581289));
#9132=CARTESIAN_POINT('Origin',(1.18440385848747,-0.07938,1.18440385848747));
#9133=CARTESIAN_POINT('Origin',(0.,-0.27783,0.));
#9134=CARTESIAN_POINT('',(0.404717578595295,-0.07938,1.65807299932179));
#9135=CARTESIAN_POINT('Origin',(0.,-0.07938,0.));
#9136=CARTESIAN_POINT('',(-0.404717578595296,-0.07938,1.65807299932179));
#9137=CARTESIAN_POINT('Ctrl Pts',(0.404717578595296,-0.0793800000000001,
1.65807299932179));
#9138=CARTESIAN_POINT('Ctrl Pts',(0.400393769631747,-0.101649918886749,
1.65912839404491));
#9139=CARTESIAN_POINT('Ctrl Pts',(0.394174530911058,-0.123823518623745,
1.66063136041479));
#9140=CARTESIAN_POINT('Ctrl Pts',(0.368536561654407,-0.192480977588835,
1.66658649961961));
#9141=CARTESIAN_POINT('Ctrl Pts',(0.341837165343982,-0.236152929235937,
1.67246562047521));
#9142=CARTESIAN_POINT('Ctrl Pts',(0.283214707341173,-0.303141259068211,
1.68332504372461));
#9143=CARTESIAN_POINT('Ctrl Pts',(0.244262842368623,-0.335108247315849,
1.68958170688653));
#9144=CARTESIAN_POINT('Ctrl Pts',(0.178166559972324,-0.373243761060364,
1.69769003172132));
#9145=CARTESIAN_POINT('Ctrl Pts',(0.143648558862931,-0.387888272594439,
1.70107730356824));
#9146=CARTESIAN_POINT('Ctrl Pts',(0.0717778861362652,-0.407041111792943,
1.70562212620408));
#9147=CARTESIAN_POINT('Ctrl Pts',(0.0344244045173309,-0.411552957311693,
1.706752));
#9148=CARTESIAN_POINT('Ctrl Pts',(-0.0344244045173315,-0.411552957311693,
1.706752));
#9149=CARTESIAN_POINT('Ctrl Pts',(-0.0717778861362658,-0.407041111792943,
1.70562212620408));
#9150=CARTESIAN_POINT('Ctrl Pts',(-0.143648558862932,-0.387888272594439,
1.70107730356824));
#9151=CARTESIAN_POINT('Ctrl Pts',(-0.178166559972325,-0.373243761060364,
1.69769003172132));
#9152=CARTESIAN_POINT('Ctrl Pts',(-0.244262842368624,-0.335108247315849,
1.68958170688653));
#9153=CARTESIAN_POINT('Ctrl Pts',(-0.283214707341173,-0.303141259068212,
1.68332504372461));
#9154=CARTESIAN_POINT('Ctrl Pts',(-0.341837165343982,-0.236152929235937,
1.67246562047521));
#9155=CARTESIAN_POINT('Ctrl Pts',(-0.368536561654408,-0.192480977588835,
1.66658649961961));
#9156=CARTESIAN_POINT('Ctrl Pts',(-0.394174530911059,-0.123823518623745,
1.66063136041479));
#9157=CARTESIAN_POINT('Ctrl Pts',(-0.400393769631748,-0.101649918886749,
1.65912839404491));
#9158=CARTESIAN_POINT('Ctrl Pts',(-0.404717578595297,-0.0793800000000001,
1.65807299932179));
#9159=CARTESIAN_POINT('',(-0.886256117232624,-0.07938,1.45861320581289));
#9160=CARTESIAN_POINT('Origin',(0.,-0.07938,0.));
#9161=CARTESIAN_POINT('',(-1.45861320581289,-0.07938,0.886256117232623));
#9162=CARTESIAN_POINT('Ctrl Pts',(-0.886256117232623,-0.0793800000000001,
1.45861320581289));
#9163=CARTESIAN_POINT('Ctrl Pts',(-0.890059788636852,-0.101649918886749,
1.45630208793976));
#9164=CARTESIAN_POINT('Ctrl Pts',(-0.895520212222106,-0.123823518623745,
1.45296717977858));
#9165=CARTESIAN_POINT('Ctrl Pts',(-0.917859913453974,-0.192480977588835,
1.43904931717599));
#9166=CARTESIAN_POINT('Ctrl Pts',(-0.940896403863071,-0.236152929235937,
1.4243271592157));
#9167=CARTESIAN_POINT('Ctrl Pts',(-0.990027513266105,-0.303141259068211,
1.39055359345152));
#9168=CARTESIAN_POINT('Ctrl Pts',(-1.02199477007745,-0.335108247315848,
1.36743459453896));
#9169=CARTESIAN_POINT('Ctrl Pts',(-1.07446535104584,-0.373243761060364,
1.32643091652006));
#9170=CARTESIAN_POINT('Ctrl Pts',(-1.10126842659597,-0.387888272594439,
1.30441816675528));
#9171=CARTESIAN_POINT('Ctrl Pts',(-1.15530234155453,-0.407041111792943,
1.25681160160691));
#9172=CARTESIAN_POINT('Ctrl Pts',(-1.18251418313119,-0.411552957311693,
1.23119764287622));
#9173=CARTESIAN_POINT('Ctrl Pts',(-1.23119764287622,-0.411552957311693,
1.18251418313119));
#9174=CARTESIAN_POINT('Ctrl Pts',(-1.25681160160691,-0.407041111792943,
1.15530234155453));
#9175=CARTESIAN_POINT('Ctrl Pts',(-1.30441816675528,-0.387888272594439,
1.10126842659597));
#9176=CARTESIAN_POINT('Ctrl Pts',(-1.32643091652006,-0.373243761060365,
1.07446535104584));
#9177=CARTESIAN_POINT('Ctrl Pts',(-1.36743459453896,-0.335108247315849,
1.02199477007745));
#9178=CARTESIAN_POINT('Ctrl Pts',(-1.39055359345152,-0.303141259068212,
0.990027513266106));
#9179=CARTESIAN_POINT('Ctrl Pts',(-1.4243271592157,-0.236152929235938,0.940896403863071));
#9180=CARTESIAN_POINT('Ctrl Pts',(-1.43904931717599,-0.192480977588836,
0.917859913453974));
#9181=CARTESIAN_POINT('Ctrl Pts',(-1.45296717977858,-0.123823518623746,
0.895520212222106));
#9182=CARTESIAN_POINT('Ctrl Pts',(-1.45630208793976,-0.101649918886749,
0.890059788636852));
#9183=CARTESIAN_POINT('Ctrl Pts',(-1.45861320581289,-0.0793800000000001,
0.886256117232623));
#9184=CARTESIAN_POINT('',(-1.65807299932179,-0.07938,0.404717578595295));
#9185=CARTESIAN_POINT('Origin',(0.,-0.07938,0.));
#9186=CARTESIAN_POINT('',(-1.706752,-0.411552957311693,2.08591827245526E-16));
#9187=CARTESIAN_POINT('Ctrl Pts',(-1.65807299932179,-0.0793800000000001,
0.404717578595296));
#9188=CARTESIAN_POINT('Ctrl Pts',(-1.65912839404491,-0.101649918886749,
0.400393769631747));
#9189=CARTESIAN_POINT('Ctrl Pts',(-1.66063136041479,-0.123823518623745,
0.394174530911058));
#9190=CARTESIAN_POINT('Ctrl Pts',(-1.66658649961961,-0.192480977588835,
0.368536561654407));
#9191=CARTESIAN_POINT('Ctrl Pts',(-1.67246562047521,-0.236152929235937,
0.341837165343982));
#9192=CARTESIAN_POINT('Ctrl Pts',(-1.68332504372461,-0.303141259068211,
0.283214707341173));
#9193=CARTESIAN_POINT('Ctrl Pts',(-1.68958170688653,-0.335108247315848,
0.244262842368623));
#9194=CARTESIAN_POINT('Ctrl Pts',(-1.69769003172132,-0.373243761060364,
0.178166559972324));
#9195=CARTESIAN_POINT('Ctrl Pts',(-1.70107730356824,-0.387888272594439,
0.143648558862931));
#9196=CARTESIAN_POINT('Ctrl Pts',(-1.70562212620408,-0.407041111792943,
0.0717778861362656));
#9197=CARTESIAN_POINT('Ctrl Pts',(-1.706752,-0.411552957311693,0.0344244045173313));
#9198=CARTESIAN_POINT('Ctrl Pts',(-1.706752,-0.411552957311693,2.08166817117217E-16));
#9199=CARTESIAN_POINT('',(-1.706752,-0.47628,2.09016837373834E-16));
#9200=CARTESIAN_POINT('',(-1.706752,-0.27783,2.09016837373834E-16));
#9201=CARTESIAN_POINT('Origin',(0.,-0.47628,0.));
#9202=CARTESIAN_POINT('',(-1.65807299932179,-0.07938,-0.404717578595296));
#9203=CARTESIAN_POINT('Ctrl Pts',(-1.706752,-0.411552957311693,2.0122792321331E-16));
#9204=CARTESIAN_POINT('Ctrl Pts',(-1.706752,-0.411552957311693,-0.0344244045173309));
#9205=CARTESIAN_POINT('Ctrl Pts',(-1.70562212620408,-0.407041111792943,
-0.0717778861362652));
#9206=CARTESIAN_POINT('Ctrl Pts',(-1.70107730356824,-0.387888272594439,
-0.143648558862931));
#9207=CARTESIAN_POINT('Ctrl Pts',(-1.69769003172132,-0.373243761060365,
-0.178166559972324));
#9208=CARTESIAN_POINT('Ctrl Pts',(-1.68958170688653,-0.335108247315849,
-0.244262842368623));
#9209=CARTESIAN_POINT('Ctrl Pts',(-1.68332504372461,-0.303141259068212,
-0.283214707341173));
#9210=CARTESIAN_POINT('Ctrl Pts',(-1.67246562047521,-0.236152929235938,
-0.341837165343982));
#9211=CARTESIAN_POINT('Ctrl Pts',(-1.66658649961961,-0.192480977588836,
-0.368536561654407));
#9212=CARTESIAN_POINT('Ctrl Pts',(-1.66063136041479,-0.123823518623745,
-0.394174530911059));
#9213=CARTESIAN_POINT('Ctrl Pts',(-1.65912839404491,-0.101649918886749,
-0.400393769631748));
#9214=CARTESIAN_POINT('Ctrl Pts',(-1.65807299932179,-0.0793800000000001,
-0.404717578595296));
#9215=CARTESIAN_POINT('',(-1.45861320581289,-0.07938,-0.886256117232623));
#9216=CARTESIAN_POINT('Origin',(0.,-0.07938,0.));
#9217=CARTESIAN_POINT('',(-0.886256117232623,-0.07938,-1.45861320581289));
#9218=CARTESIAN_POINT('Ctrl Pts',(-1.45861320581289,-0.0793800000000001,
-0.886256117232623));
#9219=CARTESIAN_POINT('Ctrl Pts',(-1.45630208793976,-0.101649918886749,
-0.890059788636852));
#9220=CARTESIAN_POINT('Ctrl Pts',(-1.45296717977858,-0.123823518623745,
-0.895520212222106));
#9221=CARTESIAN_POINT('Ctrl Pts',(-1.43904931717599,-0.192480977588835,
-0.917859913453974));
#9222=CARTESIAN_POINT('Ctrl Pts',(-1.4243271592157,-0.236152929235937,-0.940896403863072));
#9223=CARTESIAN_POINT('Ctrl Pts',(-1.39055359345152,-0.303141259068212,
-0.990027513266106));
#9224=CARTESIAN_POINT('Ctrl Pts',(-1.36743459453896,-0.335108247315849,
-1.02199477007745));
#9225=CARTESIAN_POINT('Ctrl Pts',(-1.32643091652006,-0.373243761060364,
-1.07446535104584));
#9226=CARTESIAN_POINT('Ctrl Pts',(-1.30441816675528,-0.387888272594439,
-1.10126842659597));
#9227=CARTESIAN_POINT('Ctrl Pts',(-1.25681160160691,-0.407041111792943,
-1.15530234155453));
#9228=CARTESIAN_POINT('Ctrl Pts',(-1.23119764287622,-0.411552957311693,
-1.18251418313119));
#9229=CARTESIAN_POINT('Ctrl Pts',(-1.18251418313119,-0.411552957311693,
-1.23119764287622));
#9230=CARTESIAN_POINT('Ctrl Pts',(-1.15530234155453,-0.407041111792943,
-1.25681160160691));
#9231=CARTESIAN_POINT('Ctrl Pts',(-1.10126842659597,-0.387888272594439,
-1.30441816675528));
#9232=CARTESIAN_POINT('Ctrl Pts',(-1.07446535104584,-0.373243761060364,
-1.32643091652006));
#9233=CARTESIAN_POINT('Ctrl Pts',(-1.02199477007745,-0.335108247315848,
-1.36743459453896));
#9234=CARTESIAN_POINT('Ctrl Pts',(-0.990027513266105,-0.303141259068211,
-1.39055359345152));
#9235=CARTESIAN_POINT('Ctrl Pts',(-0.940896403863071,-0.236152929235936,
-1.42432715921571));
#9236=CARTESIAN_POINT('Ctrl Pts',(-0.917859913453974,-0.192480977588835,
-1.43904931717599));
#9237=CARTESIAN_POINT('Ctrl Pts',(-0.895520212222106,-0.123823518623745,
-1.45296717977858));
#9238=CARTESIAN_POINT('Ctrl Pts',(-0.890059788636851,-0.101649918886749,
-1.45630208793976));
#9239=CARTESIAN_POINT('Ctrl Pts',(-0.886256117232623,-0.0793800000000001,
-1.45861320581289));
#9240=CARTESIAN_POINT('',(-0.404717578595295,-0.07938,-1.65807299932179));
#9241=CARTESIAN_POINT('Origin',(0.,-0.07938,0.));
#9242=CARTESIAN_POINT('',(0.404717578595296,-0.07938,-1.65807299932179));
#9243=CARTESIAN_POINT('Ctrl Pts',(-0.404717578595296,-0.0793800000000001,
-1.65807299932179));
#9244=CARTESIAN_POINT('Ctrl Pts',(-0.400393769631747,-0.101649918886749,
-1.65912839404491));
#9245=CARTESIAN_POINT('Ctrl Pts',(-0.394174530911058,-0.123823518623746,
-1.66063136041479));
#9246=CARTESIAN_POINT('Ctrl Pts',(-0.368536561654407,-0.192480977588836,
-1.66658649961961));
#9247=CARTESIAN_POINT('Ctrl Pts',(-0.341837165343982,-0.236152929235938,
-1.67246562047521));
#9248=CARTESIAN_POINT('Ctrl Pts',(-0.283214707341173,-0.303141259068212,
-1.68332504372461));
#9249=CARTESIAN_POINT('Ctrl Pts',(-0.244262842368623,-0.335108247315849,
-1.68958170688653));
#9250=CARTESIAN_POINT('Ctrl Pts',(-0.178166559972324,-0.373243761060364,
-1.69769003172132));
#9251=CARTESIAN_POINT('Ctrl Pts',(-0.143648558862931,-0.387888272594439,
-1.70107730356824));
#9252=CARTESIAN_POINT('Ctrl Pts',(-0.0717778861362653,-0.407041111792943,
-1.70562212620408));
#9253=CARTESIAN_POINT('Ctrl Pts',(-0.034424404517331,-0.411552957311693,
-1.706752));
#9254=CARTESIAN_POINT('Ctrl Pts',(0.0344244045173312,-0.411552957311693,
-1.706752));
#9255=CARTESIAN_POINT('Ctrl Pts',(0.0717778861362655,-0.407041111792943,
-1.70562212620408));
#9256=CARTESIAN_POINT('Ctrl Pts',(0.143648558862931,-0.387888272594439,
-1.70107730356824));
#9257=CARTESIAN_POINT('Ctrl Pts',(0.178166559972324,-0.373243761060364,
-1.69769003172132));
#9258=CARTESIAN_POINT('Ctrl Pts',(0.244262842368623,-0.335108247315849,
-1.68958170688653));
#9259=CARTESIAN_POINT('Ctrl Pts',(0.283214707341173,-0.303141259068212,
-1.68332504372461));
#9260=CARTESIAN_POINT('Ctrl Pts',(0.341837165343982,-0.236152929235937,
-1.67246562047521));
#9261=CARTESIAN_POINT('Ctrl Pts',(0.368536561654407,-0.192480977588835,
-1.66658649961961));
#9262=CARTESIAN_POINT('Ctrl Pts',(0.394174530911059,-0.123823518623745,
-1.66063136041479));
#9263=CARTESIAN_POINT('Ctrl Pts',(0.400393769631748,-0.101649918886749,
-1.65912839404491));
#9264=CARTESIAN_POINT('Ctrl Pts',(0.404717578595296,-0.0793800000000001,
-1.65807299932179));
#9265=CARTESIAN_POINT('',(0.886256117232623,-0.07938,-1.45861320581289));
#9266=CARTESIAN_POINT('Origin',(0.,-0.07938,0.));
#9267=CARTESIAN_POINT('',(1.45861320581289,-0.07938,-0.886256117232623));
#9268=CARTESIAN_POINT('Ctrl Pts',(0.886256117232623,-0.0793800000000001,
-1.45861320581289));
#9269=CARTESIAN_POINT('Ctrl Pts',(0.890059788636852,-0.101649918886749,
-1.45630208793976));
#9270=CARTESIAN_POINT('Ctrl Pts',(0.895520212222106,-0.123823518623745,
-1.45296717977858));
#9271=CARTESIAN_POINT('Ctrl Pts',(0.917859913453974,-0.192480977588835,
-1.43904931717599));
#9272=CARTESIAN_POINT('Ctrl Pts',(0.940896403863072,-0.236152929235937,
-1.4243271592157));
#9273=CARTESIAN_POINT('Ctrl Pts',(0.990027513266106,-0.303141259068211,
-1.39055359345152));
#9274=CARTESIAN_POINT('Ctrl Pts',(1.02199477007745,-0.335108247315849,-1.36743459453896));
#9275=CARTESIAN_POINT('Ctrl Pts',(1.07446535104584,-0.373243761060364,-1.32643091652006));
#9276=CARTESIAN_POINT('Ctrl Pts',(1.10126842659597,-0.387888272594439,-1.30441816675528));
#9277=CARTESIAN_POINT('Ctrl Pts',(1.15530234155453,-0.407041111792943,-1.25681160160691));
#9278=CARTESIAN_POINT('Ctrl Pts',(1.18251418313119,-0.411552957311693,-1.23119764287622));
#9279=CARTESIAN_POINT('Ctrl Pts',(1.23119764287622,-0.411552957311693,-1.18251418313119));
#9280=CARTESIAN_POINT('Ctrl Pts',(1.25681160160691,-0.407041111792943,-1.15530234155453));
#9281=CARTESIAN_POINT('Ctrl Pts',(1.30441816675528,-0.387888272594439,-1.10126842659597));
#9282=CARTESIAN_POINT('Ctrl Pts',(1.32643091652006,-0.373243761060364,-1.07446535104584));
#9283=CARTESIAN_POINT('Ctrl Pts',(1.36743459453896,-0.335108247315849,-1.02199477007745));
#9284=CARTESIAN_POINT('Ctrl Pts',(1.39055359345152,-0.303141259068212,-0.990027513266105));
#9285=CARTESIAN_POINT('Ctrl Pts',(1.4243271592157,-0.236152929235937,-0.940896403863071));
#9286=CARTESIAN_POINT('Ctrl Pts',(1.43904931717599,-0.192480977588835,-0.917859913453974));
#9287=CARTESIAN_POINT('Ctrl Pts',(1.45296717977858,-0.123823518623745,-0.895520212222106));
#9288=CARTESIAN_POINT('Ctrl Pts',(1.45630208793976,-0.101649918886749,-0.890059788636852));
#9289=CARTESIAN_POINT('Ctrl Pts',(1.45861320581289,-0.0793800000000001,
-0.886256117232623));
#9290=CARTESIAN_POINT('',(1.65807299932179,-0.07938,-0.404717578595296));
#9291=CARTESIAN_POINT('Origin',(0.,-0.07938,0.));
#9292=CARTESIAN_POINT('',(1.65807299932179,-0.07938,0.404717578595296));
#9293=CARTESIAN_POINT('Ctrl Pts',(1.65807299932179,-0.0793800000000001,
-0.404717578595296));
#9294=CARTESIAN_POINT('Ctrl Pts',(1.65912839404491,-0.101649918886749,-0.400393769631747));
#9295=CARTESIAN_POINT('Ctrl Pts',(1.66063136041479,-0.123823518623745,-0.394174530911058));
#9296=CARTESIAN_POINT('Ctrl Pts',(1.66658649961961,-0.192480977588835,-0.368536561654407));
#9297=CARTESIAN_POINT('Ctrl Pts',(1.67246562047521,-0.236152929235937,-0.341837165343982));
#9298=CARTESIAN_POINT('Ctrl Pts',(1.68332504372461,-0.303141259068212,-0.283214707341173));
#9299=CARTESIAN_POINT('Ctrl Pts',(1.68958170688653,-0.335108247315849,-0.244262842368623));
#9300=CARTESIAN_POINT('Ctrl Pts',(1.69769003172132,-0.373243761060364,-0.178166559972324));
#9301=CARTESIAN_POINT('Ctrl Pts',(1.70107730356824,-0.387888272594439,-0.143648558862931));
#9302=CARTESIAN_POINT('Ctrl Pts',(1.70562212620408,-0.407041111792943,-0.0717778861362655));
#9303=CARTESIAN_POINT('Ctrl Pts',(1.706752,-0.411552957311693,-0.0344244045173312));
#9304=CARTESIAN_POINT('Ctrl Pts',(1.706752,-0.411552957311693,0.0344244045173312));
#9305=CARTESIAN_POINT('Ctrl Pts',(1.70562212620408,-0.407041111792943,0.0717778861362655));
#9306=CARTESIAN_POINT('Ctrl Pts',(1.70107730356824,-0.387888272594439,0.143648558862931));
#9307=CARTESIAN_POINT('Ctrl Pts',(1.69769003172132,-0.373243761060364,0.178166559972324));
#9308=CARTESIAN_POINT('Ctrl Pts',(1.68958170688653,-0.335108247315849,0.244262842368623));
#9309=CARTESIAN_POINT('Ctrl Pts',(1.68332504372461,-0.303141259068212,0.283214707341173));
#9310=CARTESIAN_POINT('Ctrl Pts',(1.67246562047521,-0.236152929235937,0.341837165343982));
#9311=CARTESIAN_POINT('Ctrl Pts',(1.66658649961961,-0.192480977588835,0.368536561654407));
#9312=CARTESIAN_POINT('Ctrl Pts',(1.66063136041479,-0.123823518623745,0.394174530911058));
#9313=CARTESIAN_POINT('Ctrl Pts',(1.65912839404491,-0.101649918886749,0.400393769631747));
#9314=CARTESIAN_POINT('Ctrl Pts',(1.65807299932179,-0.0793800000000001,
0.404717578595296));
#9315=CARTESIAN_POINT('Origin',(0.,-0.07938,0.));
#9316=CARTESIAN_POINT('Origin',(0.,-0.07938,0.));
#9317=CARTESIAN_POINT('',(0.397005914195118,-0.07938,1.59456899932179));
#9318=CARTESIAN_POINT('Origin',(0.,-0.07938,0.));
#9319=CARTESIAN_POINT('Origin',(-3.33066907387547E-16,-0.07938,1.675));
#9320=CARTESIAN_POINT('Origin',(-3.33066907387547E-16,0.,1.675));
#9321=CARTESIAN_POINT('',(-0.397005914195118,-0.07938,1.59456899932179));
#9322=CARTESIAN_POINT('Ctrl Pts',(-0.397005914195119,-0.0793800000000001,
1.59456899932179));
#9323=CARTESIAN_POINT('Ctrl Pts',(-0.3886265584581,-0.123401821157026,1.59665523941937));
#9324=CARTESIAN_POINT('Ctrl Pts',(-0.373030350867485,-0.166543350814306,
1.60050712143809));
#9325=CARTESIAN_POINT('Ctrl Pts',(-0.333298652394954,-0.237231147975234,
1.60919314384089));
#9326=CARTESIAN_POINT('Ctrl Pts',(-0.311480544243687,-0.266264900654909,
1.61365775139403));
#9327=CARTESIAN_POINT('Ctrl Pts',(-0.261368388670537,-0.317195968905306,
1.62252828437015));
#9328=CARTESIAN_POINT('Ctrl Pts',(-0.233069203882014,-0.33909093068465,
1.62691869420078));
#9329=CARTESIAN_POINT('Ctrl Pts',(-0.174042761838764,-0.373586846396559,
1.63426473152765));
#9330=CARTESIAN_POINT('Ctrl Pts',(-0.14036578147155,-0.388086240756494,
1.63761964365402));
#9331=CARTESIAN_POINT('Ctrl Pts',(-0.0701778381840615,-0.407068917407805,
1.64212536811722));
#9332=CARTESIAN_POINT('Ctrl Pts',(-0.0336652739555918,-0.411552957311693,
1.643248));
#9333=CARTESIAN_POINT('Ctrl Pts',(0.0336652739555913,-0.411552957311693,
1.643248));
#9334=CARTESIAN_POINT('Ctrl Pts',(0.070177838184061,-0.407068917407805,
1.64212536811722));
#9335=CARTESIAN_POINT('Ctrl Pts',(0.140365781471549,-0.388086240756494,
1.63761964365402));
#9336=CARTESIAN_POINT('Ctrl Pts',(0.174042761838763,-0.373586846396559,
1.63426473152765));
#9337=CARTESIAN_POINT('Ctrl Pts',(0.233069203882014,-0.33909093068465,1.62691869420078));
#9338=CARTESIAN_POINT('Ctrl Pts',(0.261368388670536,-0.317195968905306,
1.62252828437015));
#9339=CARTESIAN_POINT('Ctrl Pts',(0.311480544243686,-0.266264900654908,
1.61365775139403));
#9340=CARTESIAN_POINT('Ctrl Pts',(0.333298652394954,-0.237231147975234,
1.60919314384089));
#9341=CARTESIAN_POINT('Ctrl Pts',(0.373030350867484,-0.166543350814306,
1.60050712143809));
#9342=CARTESIAN_POINT('Ctrl Pts',(0.388626558458099,-0.123401821157026,
1.59665523941937));
#9343=CARTESIAN_POINT('Ctrl Pts',(0.397005914195118,-0.07938,1.59456899932179));
#9344=CARTESIAN_POINT('Origin',(-3.33066907387547E-16,-0.07938,1.675));
#9345=CARTESIAN_POINT('Origin',(0.,-0.07938,0.));
#9346=CARTESIAN_POINT('',(-0.846804978391754,-0.07938,1.40825612658882));
#9347=CARTESIAN_POINT('Origin',(0.,-0.07938,0.));
#9348=CARTESIAN_POINT('Origin',(-1.18440385848747,-0.07938,1.18440385848747));
#9349=CARTESIAN_POINT('Origin',(-1.18440385848747,0.,1.18440385848747));
#9350=CARTESIAN_POINT('',(-1.40825612658882,-0.07938,0.846804978391753));
#9351=CARTESIAN_POINT('Ctrl Pts',(-1.40825612658882,-0.0793800000000001,
0.846804978391753));
#9352=CARTESIAN_POINT('Ctrl Pts',(-1.40380622184538,-0.123401821157026,
0.854205272175555));
#9353=CARTESIAN_POINT('Ctrl Pts',(-1.39550172959303,-0.166543350814306,
0.867957148219442));
#9354=CARTESIAN_POINT('Ctrl Pts',(-1.3735491215176,-0.237231147975235,0.902193646979983));
#9355=CARTESIAN_POINT('Ctrl Pts',(-1.36127834356734,-0.266264900654909,
0.920778333482565));
#9356=CARTESIAN_POINT('Ctrl Pts',(-1.33211611256184,-0.317195968905306,
0.962485392528369));
#9357=CARTESIAN_POINT('Ctrl Pts',(-1.31521005565926,-0.339090930684651,
0.985600426557816));
#9358=CARTESIAN_POINT('Ctrl Pts',(-1.27866649102984,-0.373586846396559,
1.03253285680459));
#9359=CARTESIAN_POINT('Ctrl Pts',(-1.25722555095714,-0.388086240756494,
1.05871835910697));
#9360=CARTESIAN_POINT('Ctrl Pts',(-1.2107812086231,-0.407068917407805,1.11153475808518));
#9361=CARTESIAN_POINT('Ctrl Pts',(-1.18575674747573,-0.411552957311693,
1.13814686046673));
#9362=CARTESIAN_POINT('Ctrl Pts',(-1.13814686046673,-0.411552957311693,
1.18575674747573));
#9363=CARTESIAN_POINT('Ctrl Pts',(-1.11153475808518,-0.407068917407805,
1.2107812086231));
#9364=CARTESIAN_POINT('Ctrl Pts',(-1.05871835910697,-0.388086240756494,
1.25722555095714));
#9365=CARTESIAN_POINT('Ctrl Pts',(-1.03253285680459,-0.373586846396559,
1.27866649102984));
#9366=CARTESIAN_POINT('Ctrl Pts',(-0.985600426557816,-0.33909093068465,
1.31521005565926));
#9367=CARTESIAN_POINT('Ctrl Pts',(-0.962485392528369,-0.317195968905306,
1.33211611256184));
#9368=CARTESIAN_POINT('Ctrl Pts',(-0.920778333482565,-0.266264900654908,
1.36127834356734));
#9369=CARTESIAN_POINT('Ctrl Pts',(-0.902193646979983,-0.237231147975234,
1.3735491215176));
#9370=CARTESIAN_POINT('Ctrl Pts',(-0.867957148219442,-0.166543350814306,
1.39550172959303));
#9371=CARTESIAN_POINT('Ctrl Pts',(-0.854205272175555,-0.123401821157026,
1.40380622184538));
#9372=CARTESIAN_POINT('Ctrl Pts',(-0.846804978391753,-0.0793800000000001,
1.40825612658882));
#9373=CARTESIAN_POINT('Origin',(-1.18440385848747,-0.07938,1.18440385848747));
#9374=CARTESIAN_POINT('Origin',(0.,-0.07938,0.));
#9375=CARTESIAN_POINT('',(-1.59456899932179,-0.07938,0.397005914195118));
#9376=CARTESIAN_POINT('Origin',(0.,-0.07938,0.));
#9377=CARTESIAN_POINT('Origin',(-1.675,-0.07938,-2.22044604925031E-16));
#9378=CARTESIAN_POINT('Origin',(-1.675,0.,-2.22044604925031E-16));
#9379=CARTESIAN_POINT('',(-1.59456899932179,-0.07938,-0.397005914195118));
#9380=CARTESIAN_POINT('',(-1.643248,-0.411552957311693,3.47540551556327E-18));
#9381=CARTESIAN_POINT('Ctrl Pts',(-1.59456899932179,-0.0793800000000001,
-0.397005914195119));
#9382=CARTESIAN_POINT('Ctrl Pts',(-1.59665523941937,-0.123401821157026,
-0.388626558458099));
#9383=CARTESIAN_POINT('Ctrl Pts',(-1.60050712143809,-0.166543350814306,
-0.373030350867485));
#9384=CARTESIAN_POINT('Ctrl Pts',(-1.60919314384089,-0.237231147975234,
-0.333298652394954));
#9385=CARTESIAN_POINT('Ctrl Pts',(-1.61365775139403,-0.266264900654909,
-0.311480544243686));
#9386=CARTESIAN_POINT('Ctrl Pts',(-1.62252828437015,-0.317195968905306,
-0.261368388670537));
#9387=CARTESIAN_POINT('Ctrl Pts',(-1.62691869420078,-0.33909093068465,-0.233069203882014));
#9388=CARTESIAN_POINT('Ctrl Pts',(-1.63426473152765,-0.373586846396559,
-0.174042761838764));
#9389=CARTESIAN_POINT('Ctrl Pts',(-1.63761964365402,-0.388086240756494,
-0.140365781471549));
#9390=CARTESIAN_POINT('Ctrl Pts',(-1.64212536811722,-0.407068917407805,
-0.0701778381840614));
#9391=CARTESIAN_POINT('Ctrl Pts',(-1.643248,-0.411552957311693,-0.0336652739555917));
#9392=CARTESIAN_POINT('Ctrl Pts',(-1.643248,-0.411552957311693,-2.0122792321331E-16));
#9393=CARTESIAN_POINT('Origin',(-1.675,-0.07938,-2.22044604925031E-16));
#9394=CARTESIAN_POINT('Ctrl Pts',(-1.643248,-0.411552957311693,-1.94289029309402E-16));
#9395=CARTESIAN_POINT('Ctrl Pts',(-1.643248,-0.411552957311693,0.0336652739555913));
#9396=CARTESIAN_POINT('Ctrl Pts',(-1.64212536811722,-0.407068917407805,
0.0701778381840609));
#9397=CARTESIAN_POINT('Ctrl Pts',(-1.63761964365402,-0.388086240756494,
0.140365781471549));
#9398=CARTESIAN_POINT('Ctrl Pts',(-1.63426473152765,-0.373586846396559,
0.174042761838763));
#9399=CARTESIAN_POINT('Ctrl Pts',(-1.62691869420078,-0.33909093068465,0.233069203882014));
#9400=CARTESIAN_POINT('Ctrl Pts',(-1.62252828437015,-0.317195968905306,
0.261368388670536));
#9401=CARTESIAN_POINT('Ctrl Pts',(-1.61365775139403,-0.266264900654909,
0.311480544243686));
#9402=CARTESIAN_POINT('Ctrl Pts',(-1.60919314384089,-0.237231147975235,
0.333298652394954));
#9403=CARTESIAN_POINT('Ctrl Pts',(-1.60050712143809,-0.166543350814306,
0.373030350867484));
#9404=CARTESIAN_POINT('Ctrl Pts',(-1.59665523941937,-0.123401821157026,
0.388626558458099));
#9405=CARTESIAN_POINT('Ctrl Pts',(-1.59456899932179,-0.0793800000000001,
0.397005914195118));
#9406=CARTESIAN_POINT('Origin',(0.,-0.07938,0.));
#9407=CARTESIAN_POINT('',(-1.40825612658882,-0.07938,-0.846804978391753));
#9408=CARTESIAN_POINT('Origin',(0.,-0.07938,0.));
#9409=CARTESIAN_POINT('Origin',(-1.18440385848747,-0.07938,-1.18440385848747));
#9410=CARTESIAN_POINT('Origin',(-1.18440385848747,0.,-1.18440385848747));
#9411=CARTESIAN_POINT('',(-0.846804978391753,-0.07938,-1.40825612658882));
#9412=CARTESIAN_POINT('Ctrl Pts',(-0.846804978391753,-0.0793800000000001,
-1.40825612658882));
#9413=CARTESIAN_POINT('Ctrl Pts',(-0.854205272175555,-0.123401821157026,
-1.40380622184538));
#9414=CARTESIAN_POINT('Ctrl Pts',(-0.867957148219442,-0.166543350814306,
-1.39550172959303));
#9415=CARTESIAN_POINT('Ctrl Pts',(-0.902193646979982,-0.237231147975234,
-1.3735491215176));
#9416=CARTESIAN_POINT('Ctrl Pts',(-0.920778333482564,-0.266264900654908,
-1.36127834356734));
#9417=CARTESIAN_POINT('Ctrl Pts',(-0.962485392528368,-0.317195968905306,
-1.33211611256184));
#9418=CARTESIAN_POINT('Ctrl Pts',(-0.985600426557816,-0.33909093068465,
-1.31521005565926));
#9419=CARTESIAN_POINT('Ctrl Pts',(-1.03253285680459,-0.373586846396559,
-1.27866649102984));
#9420=CARTESIAN_POINT('Ctrl Pts',(-1.05871835910697,-0.388086240756494,
-1.25722555095714));
#9421=CARTESIAN_POINT('Ctrl Pts',(-1.11153475808518,-0.407068917407805,
-1.2107812086231));
#9422=CARTESIAN_POINT('Ctrl Pts',(-1.13814686046673,-0.411552957311693,
-1.18575674747573));
#9423=CARTESIAN_POINT('Ctrl Pts',(-1.18575674747573,-0.411552957311693,
-1.13814686046673));
#9424=CARTESIAN_POINT('Ctrl Pts',(-1.2107812086231,-0.407068917407805,-1.11153475808518));
#9425=CARTESIAN_POINT('Ctrl Pts',(-1.25722555095714,-0.388086240756494,
-1.05871835910697));
#9426=CARTESIAN_POINT('Ctrl Pts',(-1.27866649102984,-0.373586846396559,
-1.03253285680459));
#9427=CARTESIAN_POINT('Ctrl Pts',(-1.31521005565926,-0.33909093068465,-0.985600426557816));
#9428=CARTESIAN_POINT('Ctrl Pts',(-1.33211611256184,-0.317195968905306,
-0.962485392528369));
#9429=CARTESIAN_POINT('Ctrl Pts',(-1.36127834356734,-0.266264900654909,
-0.920778333482565));
#9430=CARTESIAN_POINT('Ctrl Pts',(-1.3735491215176,-0.237231147975234,-0.902193646979983));
#9431=CARTESIAN_POINT('Ctrl Pts',(-1.39550172959303,-0.166543350814306,
-0.867957148219442));
#9432=CARTESIAN_POINT('Ctrl Pts',(-1.40380622184538,-0.123401821157026,
-0.854205272175555));
#9433=CARTESIAN_POINT('Ctrl Pts',(-1.40825612658882,-0.07938,-0.846804978391753));
#9434=CARTESIAN_POINT('Origin',(-1.18440385848747,-0.07938,-1.18440385848747));
#9435=CARTESIAN_POINT('Origin',(0.,-0.07938,0.));
#9436=CARTESIAN_POINT('',(-0.397005914195118,-0.07938,-1.59456899932179));
#9437=CARTESIAN_POINT('Origin',(0.,-0.07938,0.));
#9438=CARTESIAN_POINT('Origin',(1.11022302462516E-16,-0.07938,-1.675));
#9439=CARTESIAN_POINT('Origin',(1.11022302462516E-16,0.,-1.675));
#9440=CARTESIAN_POINT('',(0.397005914195118,-0.07938,-1.59456899932179));
#9441=CARTESIAN_POINT('Ctrl Pts',(0.397005914195119,-0.0793800000000001,
-1.59456899932179));
#9442=CARTESIAN_POINT('Ctrl Pts',(0.388626558458099,-0.123401821157026,
-1.59665523941937));
#9443=CARTESIAN_POINT('Ctrl Pts',(0.373030350867485,-0.166543350814306,
-1.60050712143809));
#9444=CARTESIAN_POINT('Ctrl Pts',(0.333298652394954,-0.237231147975234,
-1.60919314384089));
#9445=CARTESIAN_POINT('Ctrl Pts',(0.311480544243686,-0.266264900654909,
-1.61365775139403));
#9446=CARTESIAN_POINT('Ctrl Pts',(0.261368388670537,-0.317195968905306,
-1.62252828437015));
#9447=CARTESIAN_POINT('Ctrl Pts',(0.233069203882014,-0.33909093068465,-1.62691869420078));
#9448=CARTESIAN_POINT('Ctrl Pts',(0.174042761838763,-0.373586846396559,
-1.63426473152765));
#9449=CARTESIAN_POINT('Ctrl Pts',(0.140365781471549,-0.388086240756494,
-1.63761964365402));
#9450=CARTESIAN_POINT('Ctrl Pts',(0.0701778381840612,-0.407068917407805,
-1.64212536811722));
#9451=CARTESIAN_POINT('Ctrl Pts',(0.0336652739555916,-0.411552957311693,
-1.643248));
#9452=CARTESIAN_POINT('Ctrl Pts',(-0.0336652739555915,-0.411552957311693,
-1.643248));
#9453=CARTESIAN_POINT('Ctrl Pts',(-0.0701778381840612,-0.407068917407805,
-1.64212536811722));
#9454=CARTESIAN_POINT('Ctrl Pts',(-0.140365781471549,-0.388086240756494,
-1.63761964365402));
#9455=CARTESIAN_POINT('Ctrl Pts',(-0.174042761838764,-0.373586846396559,
-1.63426473152765));
#9456=CARTESIAN_POINT('Ctrl Pts',(-0.233069203882014,-0.33909093068465,
-1.62691869420078));
#9457=CARTESIAN_POINT('Ctrl Pts',(-0.261368388670536,-0.317195968905306,
-1.62252828437015));
#9458=CARTESIAN_POINT('Ctrl Pts',(-0.311480544243686,-0.266264900654908,
-1.61365775139403));
#9459=CARTESIAN_POINT('Ctrl Pts',(-0.333298652394954,-0.237231147975234,
-1.60919314384089));
#9460=CARTESIAN_POINT('Ctrl Pts',(-0.373030350867485,-0.166543350814306,
-1.60050712143809));
#9461=CARTESIAN_POINT('Ctrl Pts',(-0.388626558458099,-0.123401821157026,
-1.59665523941937));
#9462=CARTESIAN_POINT('Ctrl Pts',(-0.397005914195118,-0.07938,-1.59456899932179));
#9463=CARTESIAN_POINT('Origin',(1.11022302462516E-16,-0.07938,-1.675));
#9464=CARTESIAN_POINT('Origin',(0.,-0.07938,0.));
#9465=CARTESIAN_POINT('',(0.846804978391753,-0.07938,-1.40825612658882));
#9466=CARTESIAN_POINT('Origin',(0.,-0.07938,0.));
#9467=CARTESIAN_POINT('Origin',(1.18440385848747,-0.07938,-1.18440385848747));
#9468=CARTESIAN_POINT('Origin',(1.18440385848747,0.,-1.18440385848747));
#9469=CARTESIAN_POINT('',(1.40825612658882,-0.07938,-0.846804978391753));
#9470=CARTESIAN_POINT('Ctrl Pts',(1.40825612658882,-0.0793800000000001,
-0.846804978391753));
#9471=CARTESIAN_POINT('Ctrl Pts',(1.40380622184538,-0.123401821157026,-0.854205272175555));
#9472=CARTESIAN_POINT('Ctrl Pts',(1.39550172959303,-0.166543350814306,-0.867957148219442));
#9473=CARTESIAN_POINT('Ctrl Pts',(1.3735491215176,-0.237231147975234,-0.902193646979983));
#9474=CARTESIAN_POINT('Ctrl Pts',(1.36127834356734,-0.266264900654908,-0.920778333482565));
#9475=CARTESIAN_POINT('Ctrl Pts',(1.33211611256184,-0.317195968905306,-0.962485392528369));
#9476=CARTESIAN_POINT('Ctrl Pts',(1.31521005565926,-0.33909093068465,-0.985600426557816));
#9477=CARTESIAN_POINT('Ctrl Pts',(1.27866649102984,-0.373586846396559,-1.03253285680459));
#9478=CARTESIAN_POINT('Ctrl Pts',(1.25722555095714,-0.388086240756494,-1.05871835910697));
#9479=CARTESIAN_POINT('Ctrl Pts',(1.2107812086231,-0.407068917407805,-1.11153475808518));
#9480=CARTESIAN_POINT('Ctrl Pts',(1.18575674747573,-0.411552957311693,-1.13814686046673));
#9481=CARTESIAN_POINT('Ctrl Pts',(1.13814686046673,-0.411552957311693,-1.18575674747573));
#9482=CARTESIAN_POINT('Ctrl Pts',(1.11153475808518,-0.407068917407805,-1.2107812086231));
#9483=CARTESIAN_POINT('Ctrl Pts',(1.05871835910697,-0.388086240756494,-1.25722555095714));
#9484=CARTESIAN_POINT('Ctrl Pts',(1.03253285680459,-0.373586846396559,-1.27866649102984));
#9485=CARTESIAN_POINT('Ctrl Pts',(0.985600426557816,-0.33909093068465,-1.31521005565926));
#9486=CARTESIAN_POINT('Ctrl Pts',(0.962485392528369,-0.317195968905306,
-1.33211611256184));
#9487=CARTESIAN_POINT('Ctrl Pts',(0.920778333482565,-0.266264900654909,
-1.36127834356734));
#9488=CARTESIAN_POINT('Ctrl Pts',(0.902193646979983,-0.237231147975234,
-1.3735491215176));
#9489=CARTESIAN_POINT('Ctrl Pts',(0.867957148219442,-0.166543350814306,
-1.39550172959303));
#9490=CARTESIAN_POINT('Ctrl Pts',(0.854205272175555,-0.123401821157026,
-1.40380622184538));
#9491=CARTESIAN_POINT('Ctrl Pts',(0.846804978391753,-0.0793800000000001,
-1.40825612658882));
#9492=CARTESIAN_POINT('Origin',(1.18440385848747,-0.07938,-1.18440385848747));
#9493=CARTESIAN_POINT('Origin',(0.,-0.27783,0.));
#9494=CARTESIAN_POINT('',(-1.643248,-0.47628,2.01239840340529E-16));
#9495=CARTESIAN_POINT('Origin',(0.,-0.47628,0.));
#9496=CARTESIAN_POINT('',(-1.643248,-0.27783,2.01239840340529E-16));
#9497=CARTESIAN_POINT('',(1.59456899932179,-0.07938,0.397005914195118));
#9498=CARTESIAN_POINT('Origin',(0.,-0.07938,0.));
#9499=CARTESIAN_POINT('',(1.59456899932179,-0.07938,-0.397005914195118));
#9500=CARTESIAN_POINT('Ctrl Pts',(1.59456899932179,-0.0793800000000001,
0.397005914195118));
#9501=CARTESIAN_POINT('Ctrl Pts',(1.59665523941937,-0.123401821157026,0.388626558458099));
#9502=CARTESIAN_POINT('Ctrl Pts',(1.60050712143809,-0.166543350814306,0.373030350867485));
#9503=CARTESIAN_POINT('Ctrl Pts',(1.60919314384089,-0.237231147975234,0.333298652394954));
#9504=CARTESIAN_POINT('Ctrl Pts',(1.61365775139403,-0.266264900654909,0.311480544243686));
#9505=CARTESIAN_POINT('Ctrl Pts',(1.62252828437015,-0.317195968905306,0.261368388670537));
#9506=CARTESIAN_POINT('Ctrl Pts',(1.62691869420078,-0.33909093068465,0.233069203882014));
#9507=CARTESIAN_POINT('Ctrl Pts',(1.63426473152765,-0.373586846396559,0.174042761838764));
#9508=CARTESIAN_POINT('Ctrl Pts',(1.63761964365402,-0.388086240756494,0.140365781471549));
#9509=CARTESIAN_POINT('Ctrl Pts',(1.64212536811722,-0.407068917407805,0.0701778381840612));
#9510=CARTESIAN_POINT('Ctrl Pts',(1.643248,-0.411552957311693,0.0336652739555916));
#9511=CARTESIAN_POINT('Ctrl Pts',(1.643248,-0.411552957311693,-0.0336652739555916));
#9512=CARTESIAN_POINT('Ctrl Pts',(1.64212536811722,-0.407068917407805,-0.0701778381840612));
#9513=CARTESIAN_POINT('Ctrl Pts',(1.63761964365402,-0.388086240756494,-0.140365781471549));
#9514=CARTESIAN_POINT('Ctrl Pts',(1.63426473152765,-0.373586846396559,-0.174042761838764));
#9515=CARTESIAN_POINT('Ctrl Pts',(1.62691869420078,-0.33909093068465,-0.233069203882014));
#9516=CARTESIAN_POINT('Ctrl Pts',(1.62252828437015,-0.317195968905306,-0.261368388670537));
#9517=CARTESIAN_POINT('Ctrl Pts',(1.61365775139403,-0.266264900654909,-0.311480544243686));
#9518=CARTESIAN_POINT('Ctrl Pts',(1.60919314384089,-0.237231147975234,-0.333298652394954));
#9519=CARTESIAN_POINT('Ctrl Pts',(1.60050712143809,-0.166543350814306,-0.373030350867485));
#9520=CARTESIAN_POINT('Ctrl Pts',(1.59665523941937,-0.123401821157026,-0.388626558458099));
#9521=CARTESIAN_POINT('Ctrl Pts',(1.59456899932179,-0.07938,-0.397005914195118));
#9522=CARTESIAN_POINT('Origin',(0.,-0.07938,0.));
#9523=CARTESIAN_POINT('Origin',(0.,-0.07938,0.));
#9524=CARTESIAN_POINT('Origin',(1.675,-0.07938,0.));
#9525=CARTESIAN_POINT('Origin',(1.675,0.,0.));
#9526=CARTESIAN_POINT('Origin',(1.675,-0.07938,0.));
#9527=CARTESIAN_POINT('Origin',(0.,-0.47628,0.));
#9528=CARTESIAN_POINT('Origin',(0.,-0.07938,0.));
#10924=UNCERTAINTY_MEASURE_WITH_UNIT(LENGTH_MEASURE(0.001),#10964,
'DISTANCE_ACCURACY_VALUE',
'Maximum model space distance between geometric entities at asserted c
onnectivities');
#10936=UNCERTAINTY_MEASURE_WITH_UNIT(LENGTH_MEASURE(0.001),#10964,
'DISTANCE_ACCURACY_VALUE',
'Maximum model space distance between geometric entities at asserted c
onnectivities');
#10951=(
GEOMETRIC_REPRESENTATION_CONTEXT(3)
GLOBAL_UNCERTAINTY_ASSIGNED_CONTEXT((#10924))
GLOBAL_UNIT_ASSIGNED_CONTEXT((#10964,#10966,#10967))
REPRESENTATION_CONTEXT('','3D')
);
#10963=(
GEOMETRIC_REPRESENTATION_CONTEXT(3)
GLOBAL_UNCERTAINTY_ASSIGNED_CONTEXT((#10936))
GLOBAL_UNIT_ASSIGNED_CONTEXT((#10964,#10966,#10967))
REPRESENTATION_CONTEXT('','3D')
);
#10964=(
LENGTH_UNIT()
NAMED_UNIT(*)
SI_UNIT(.CENTI.,.METRE.)
);
#10966=(
NAMED_UNIT(*)
PLANE_ANGLE_UNIT()
SI_UNIT($,.RADIAN.)
);
#10967=(
NAMED_UNIT(*)
SI_UNIT($,.STERADIAN.)
SOLID_ANGLE_UNIT()
);
#10982=SHAPE_DEFINITION_REPRESENTATION(#11008,#11071);
#11008=PRODUCT_DEFINITION_SHAPE('',$,#11098);
#11071=SHAPE_REPRESENTATION('',(#6169),#10951);
#11083=PRODUCT_DEFINITION_CONTEXT('part definition',#11163,'design');
#11098=PRODUCT_DEFINITION('Cage','Cage',#11124,#11083);
#11124=PRODUCT_DEFINITION_FORMATION('',$,#11179);
#11163=APPLICATION_CONTEXT(
'Core Data for Automotive Mechanical Design Process');
#11164=PRODUCT_CONTEXT('part definition',#11163,'mechanical');
#11179=PRODUCT('Cage','Cage','Cage',(#11164));
#11247=COLOUR_RGB('Grey',0.48,0.52,0.57);
#11248=FILL_AREA_STYLE_COLOUR('',#11247);
#11249=FILL_AREA_STYLE('',(#11248));
#11250=SURFACE_STYLE_FILL_AREA(#11249);
#11251=SURFACE_SIDE_STYLE('',(#11250));
#11252=SURFACE_STYLE_USAGE(.BOTH.,#11251);
#11253=PRESENTATION_STYLE_ASSIGNMENT((#11252));
ENDSEC;
END-ISO-10303-21;
